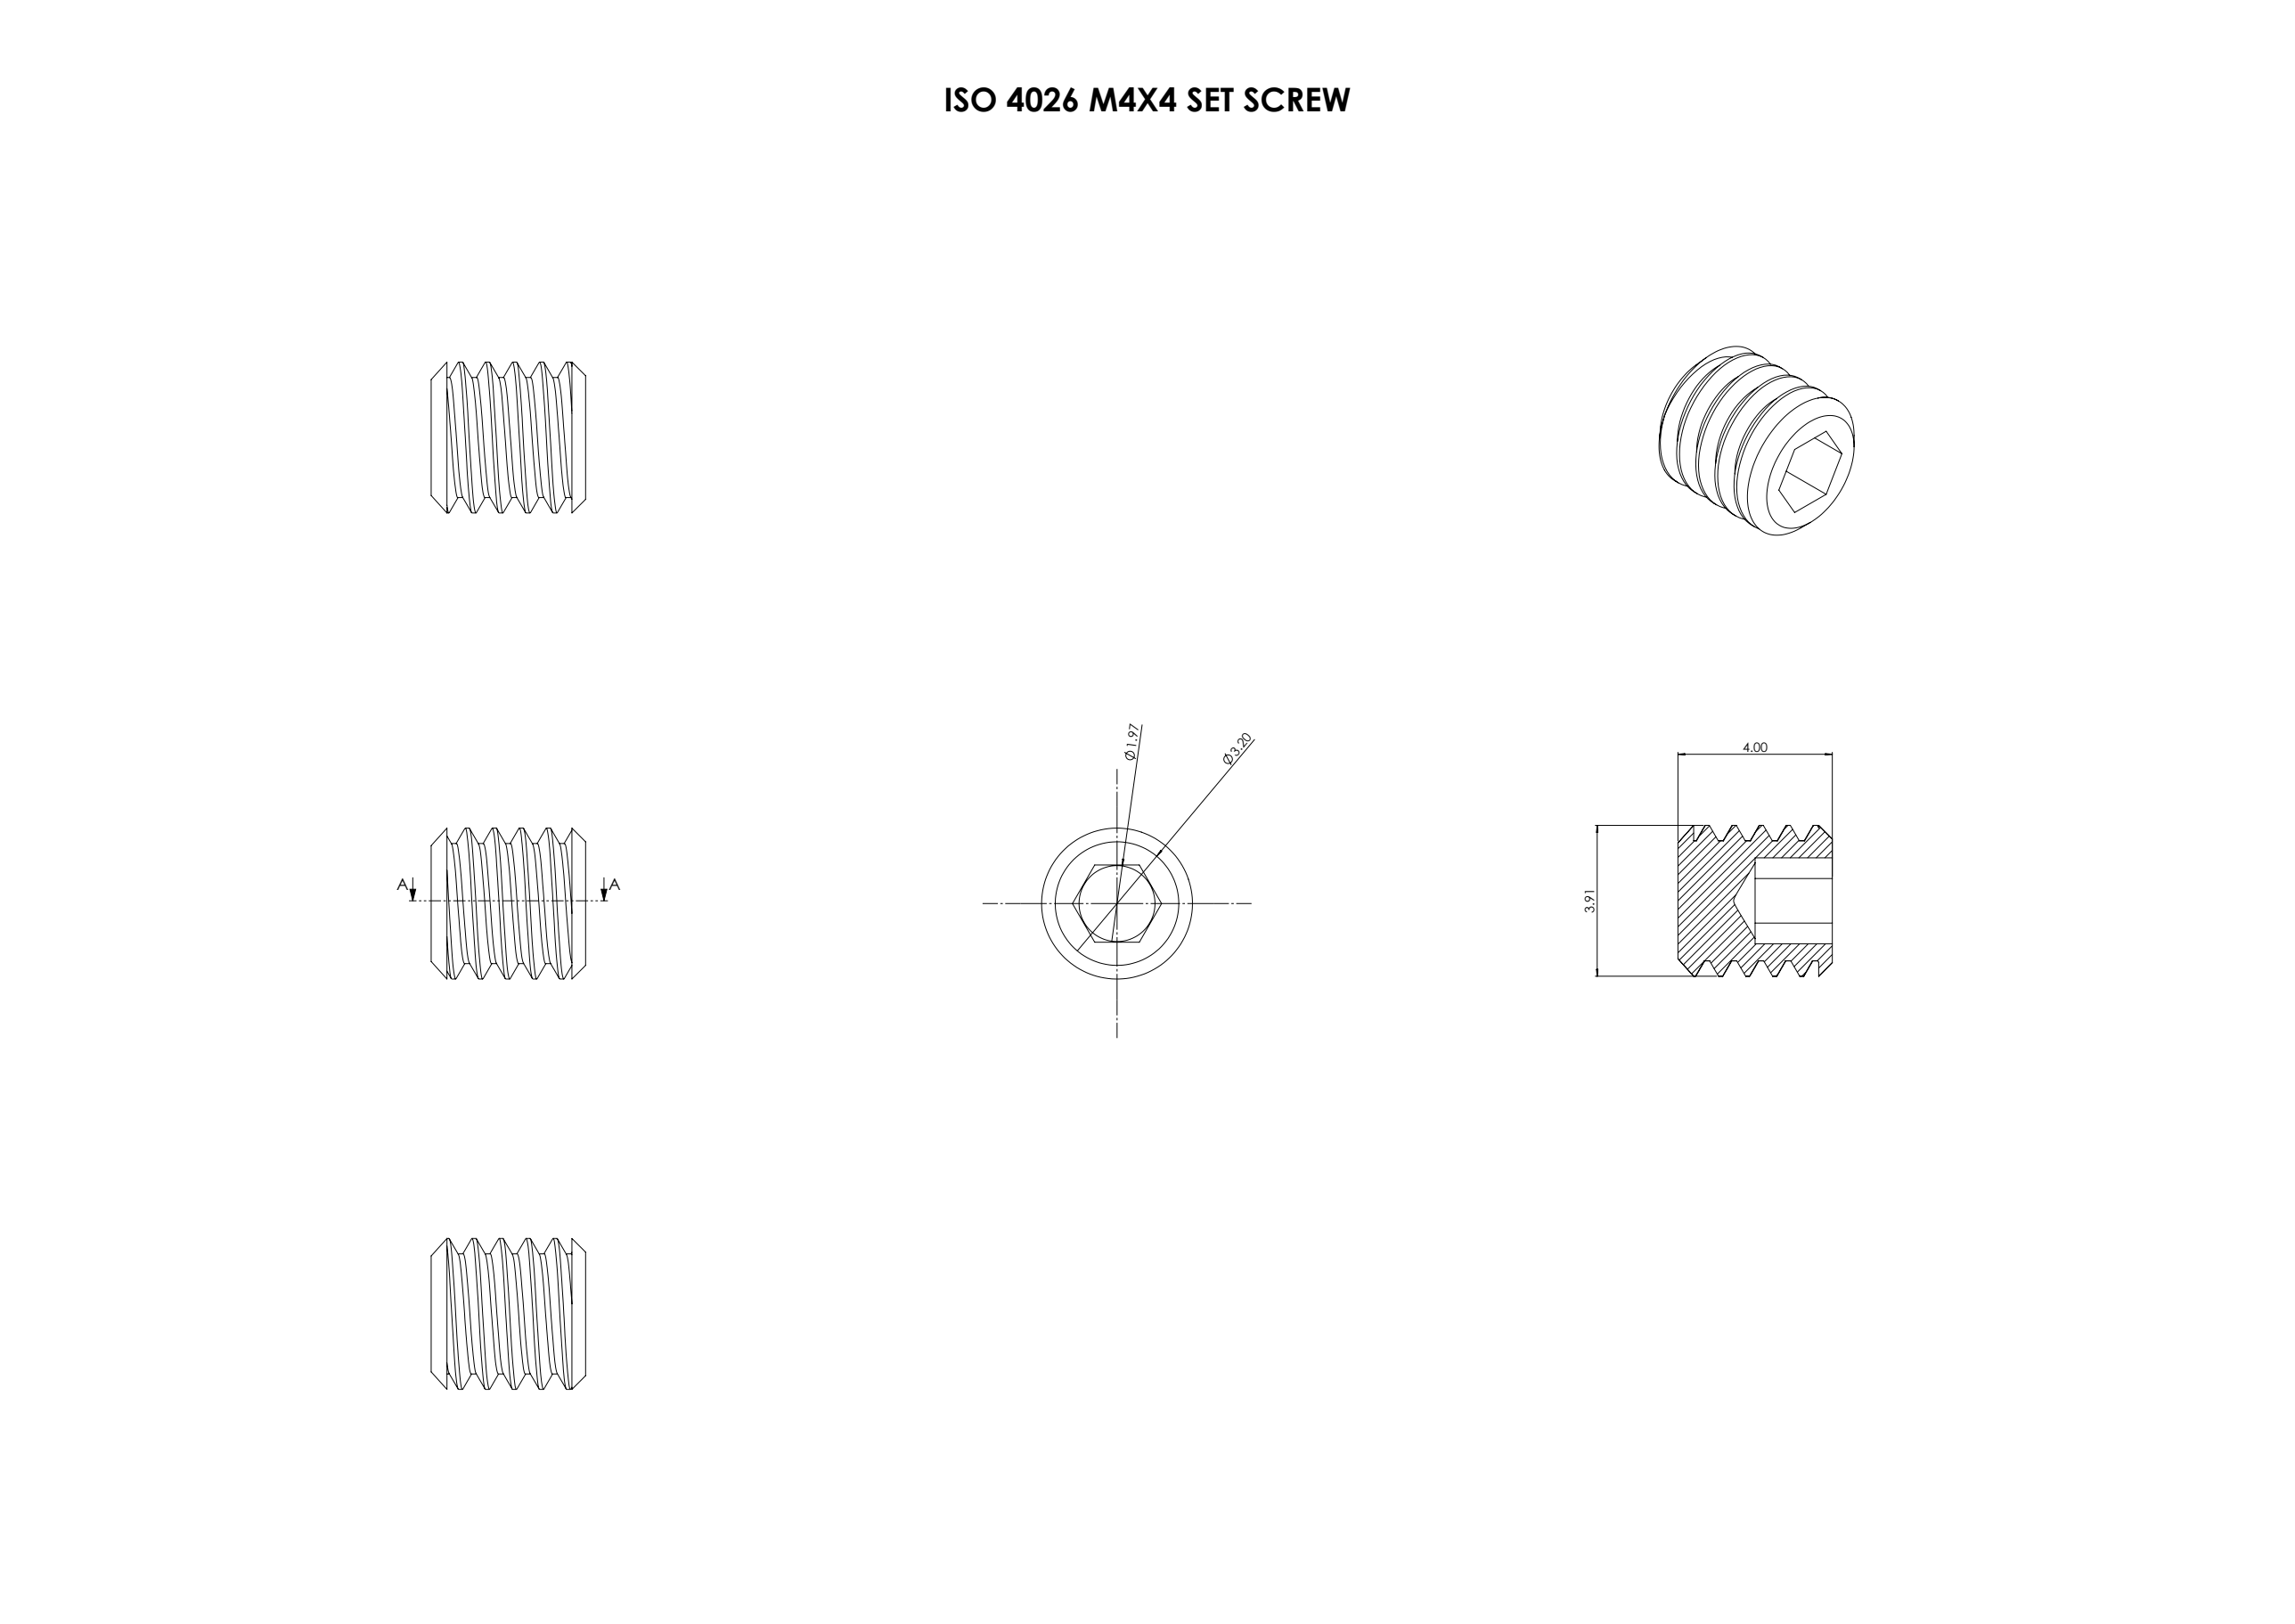
ISO-10303-21;
HEADER;
/* Generated by software containing ST-Developer
 * from STEP Tools, Inc. (www.steptools.com) 
 */

FILE_DESCRIPTION(
/* description */ (''),
/* implementation_level */ '2;1');

FILE_NAME(
/* name */ '09_ISO_4026_M4x4_Set_Screw.step',
/* time_stamp */ '2026-10-11T09:12:28-07:00',
/* author */ (''),
/* organization */ (''),
/* preprocessor_version */ 'ST-DEVELOPER v20.2',
/* originating_system */ 'Autodesk Translation Framework v15.15.0.0',
/* authorisation */ '');

FILE_SCHEMA (('AUTOMOTIVE_DESIGN { 1 0 10303 214 3 1 1 }'));
ENDSEC;

DATA;
#10=MECHANICAL_DESIGN_GEOMETRIC_PRESENTATION_REPRESENTATION('',(#655),#23254);
#173=B_SPLINE_SURFACE_WITH_KNOTS('',3,3,((#22595,#22596,#22597,#22598,#22599,
#22600,#22601,#22602,#22603,#22604,#22605,#22606,#22607,#22608,#22609,#22610,
#22611,#22612,#22613,#22614,#22615,#22616,#22617,#22618,#22619,#22620,#22621,
#22622,#22623,#22624,#22625,#22626,#22627,#22628,#22629),(#22630,#22631,
#22632,#22633,#22634,#22635,#22636,#22637,#22638,#22639,#22640,#22641,#22642,
#22643,#22644,#22645,#22646,#22647,#22648,#22649,#22650,#22651,#22652,#22653,
#22654,#22655,#22656,#22657,#22658,#22659,#22660,#22661,#22662,#22663,#22664),
(#22665,#22666,#22667,#22668,#22669,#22670,#22671,#22672,#22673,#22674,
#22675,#22676,#22677,#22678,#22679,#22680,#22681,#22682,#22683,#22684,#22685,
#22686,#22687,#22688,#22689,#22690,#22691,#22692,#22693,#22694,#22695,#22696,
#22697,#22698,#22699),(#22700,#22701,#22702,#22703,#22704,#22705,#22706,
#22707,#22708,#22709,#22710,#22711,#22712,#22713,#22714,#22715,#22716,#22717,
#22718,#22719,#22720,#22721,#22722,#22723,#22724,#22725,#22726,#22727,#22728,
#22729,#22730,#22731,#22732,#22733,#22734)),.UNSPECIFIED.,.F.,.F.,.F.,(4,
4),(4,1,1,1,1,1,1,1,1,1,1,1,1,1,1,1,1,1,1,1,1,1,1,1,1,1,1,1,1,1,1,1,4),
(0.,0.0460148164544132),(8.31058692273979,9.28321112839862,10.2558353340575,
11.2284595397163,12.2010837453751,13.173707951034,14.1463321566928,15.1189563623516,
16.0915805680104,17.0642047736693,18.0368289793281,19.0094531849869,19.9820773906458,
20.9547015963046,21.9273258019634,22.8999500076223,23.8725742132811,24.8451984189399,
25.8178226245988,26.7904468302576,27.7630710359164,28.7356952415753,29.7083194472341,
30.6809436528929,31.6535678585518,32.6261920642106,33.5988162698694,34.5714404755283,
35.5440646811871,36.5166888868459,37.4893130925048,38.4619372981636,39.4345615038224),
 .UNSPECIFIED.);
#174=B_SPLINE_SURFACE_WITH_KNOTS('',3,3,((#22949,#22950,#22951,#22952,#22953,
#22954,#22955,#22956,#22957,#22958,#22959,#22960,#22961,#22962,#22963,#22964,
#22965,#22966,#22967,#22968,#22969,#22970,#22971,#22972,#22973,#22974,#22975,
#22976,#22977,#22978,#22979,#22980,#22981,#22982,#22983),(#22984,#22985,
#22986,#22987,#22988,#22989,#22990,#22991,#22992,#22993,#22994,#22995,#22996,
#22997,#22998,#22999,#23000,#23001,#23002,#23003,#23004,#23005,#23006,#23007,
#23008,#23009,#23010,#23011,#23012,#23013,#23014,#23015,#23016,#23017,#23018),
(#23019,#23020,#23021,#23022,#23023,#23024,#23025,#23026,#23027,#23028,
#23029,#23030,#23031,#23032,#23033,#23034,#23035,#23036,#23037,#23038,#23039,
#23040,#23041,#23042,#23043,#23044,#23045,#23046,#23047,#23048,#23049,#23050,
#23051,#23052,#23053),(#23054,#23055,#23056,#23057,#23058,#23059,#23060,
#23061,#23062,#23063,#23064,#23065,#23066,#23067,#23068,#23069,#23070,#23071,
#23072,#23073,#23074,#23075,#23076,#23077,#23078,#23079,#23080,#23081,#23082,
#23083,#23084,#23085,#23086,#23087,#23088)),.UNSPECIFIED.,.F.,.F.,.F.,(4,
4),(4,1,1,1,1,1,1,1,1,1,1,1,1,1,1,1,1,1,1,1,1,1,1,1,1,1,1,1,1,1,1,1,4),
(0.,0.0460148164544132),(11.6154215191107,12.5880457247695,13.5606699304283,
14.5332941360872,15.505918341746,16.4785425474048,17.4511667530637,18.4237909587225,
19.3964151643813,20.3690393700402,21.341663575699,22.3142877813578,23.2869119870167,
24.2595361926755,25.2321603983343,26.2047846039932,27.177408809652,28.1500330153108,
29.1226572209696,30.0952814266285,31.0679056322873,32.0405298379462,33.013154043605,
33.9857782492638,34.9584024549226,35.9310266605815,36.9036508662403,37.8762750718991,
38.848899277558,39.8215234832168,40.7941476888756,41.7667718945345,42.7393961001933),
 .UNSPECIFIED.);
#601=B_SPLINE_CURVE_WITH_KNOTS('',3,(#22093,#22094,#22095,#22096,#22097,
#22098,#22099,#22100,#22101,#22102),.UNSPECIFIED.,.F.,.F.,(4,3,3,4),(-4.0925417488383,
-3.89049682263533,-2.9178726169765,-2.0651401332781),.UNSPECIFIED.);
#602=B_SPLINE_CURVE_WITH_KNOTS('',3,(#22105,#22106,#22107,#22108,#22109,
#22110,#22111),.UNSPECIFIED.,.F.,.F.,(4,3,4),(0.,0.972624205658834,1.11419103802959),
 .UNSPECIFIED.);
#603=B_SPLINE_CURVE_WITH_KNOTS('',3,(#22116,#22117,#22118,#22119,#22120,
#22121,#22122,#22123,#22124,#22125,#22126,#22127,#22128,#22129,#22130,#22131,
#22132,#22133,#22134,#22135,#22136,#22137),.UNSPECIFIED.,.F.,.F.,(4,3,3,
3,3,3,3,4),(-10.3757270560179,-9.72624205658833,-8.7536178509295,-7.78099364527067,
-6.80836943961183,-5.835745233953,-4.86312102829416,-4.0925417488383),
 .UNSPECIFIED.);
#604=B_SPLINE_CURVE_WITH_KNOTS('',3,(#22138,#22139,#22140,#22141,#22142,
#22143,#22144,#22145,#22146,#22147,#22148,#22149,#22150,#22151,#22152,#22153,
#22154,#22155,#22156,#22157,#22158,#22159),.UNSPECIFIED.,.F.,.F.,(4,3,3,
3,3,3,3,4),(1.11419103802959,1.94524841131767,2.9178726169765,3.89049682263533,
4.86312102829416,5.835745233953,6.80836943961183,7.39737634520917),
 .UNSPECIFIED.);
#605=B_SPLINE_CURVE_WITH_KNOTS('',3,(#22164,#22165,#22166,#22167,#22168,
#22169,#22170,#22171,#22172,#22173,#22174,#22175,#22176,#22177,#22178,#22179,
#22180,#22181,#22182,#22183,#22184,#22185,#22186,#22187,#22188),
 .UNSPECIFIED.,.F.,.F.,(4,3,3,3,3,3,3,3,4),(-16.6589123631975,-16.5346114962002,
-15.5619872905413,-14.5893630848825,-13.6167388792237,-12.6441146735648,
-11.671490467906,-10.6988662622472,-10.3757270560179),.UNSPECIFIED.);
#606=B_SPLINE_CURVE_WITH_KNOTS('',3,(#22189,#22190,#22191,#22192,#22193,
#22194,#22195,#22196,#22197,#22198,#22199,#22200,#22201,#22202,#22203,#22204,
#22205,#22206,#22207,#22208,#22209,#22210,#22211,#22212,#22213),
 .UNSPECIFIED.,.F.,.F.,(4,3,3,3,3,3,3,3,4),(7.39737634520917,7.78099364527067,
8.7536178509295,9.72624205658833,10.6988662622472,11.671490467906,12.6441146735648,
13.6167388792237,13.6805616523888),.UNSPECIFIED.);
#607=B_SPLINE_CURVE_WITH_KNOTS('',3,(#22218,#22219,#22220,#22221,#22222,
#22223,#22224,#22225,#22226,#22227,#22228,#22229,#22230,#22231,#22232,#22233,
#22234,#22235,#22236,#22237,#22238,#22239),.UNSPECIFIED.,.F.,.F.,(4,3,3,
3,3,3,3,4),(-22.9420976703771,-22.3703567301532,-21.3977325244943,-20.4251083188355,
-19.4524841131767,-18.4798599075178,-17.507235701859,-16.6589123631975),
 .UNSPECIFIED.);
#608=B_SPLINE_CURVE_WITH_KNOTS('',3,(#22240,#22241,#22242,#22243,#22244,
#22245,#22246,#22247,#22248,#22249,#22250,#22251,#22252,#22253,#22254,#22255,
#22256,#22257,#22258,#22259,#22260,#22261),.UNSPECIFIED.,.F.,.F.,(4,3,3,
3,3,3,3,4),(13.6805616523888,14.5893630848825,15.5619872905413,16.5346114962002,
17.507235701859,18.4798599075178,19.4524841131767,19.9637469595683),
 .UNSPECIFIED.);
#609=B_SPLINE_CURVE_WITH_KNOTS('',3,(#22266,#22267,#22268,#22269,#22270,
#22271,#22272,#22273,#22274,#22275,#22276,#22277,#22278,#22279,#22280,#22281,
#22282,#22283,#22284,#22285,#22286,#22287,#22288,#22289,#22290),
 .UNSPECIFIED.,.F.,.F.,(4,3,3,3,3,3,3,3,4),(-29.2252829775566,-29.178726169765,
-28.2061019641061,-27.2334777584473,-26.2608535527885,-25.2882293471297,
-24.3156051414708,-23.342980935812,-22.9420976703771),.UNSPECIFIED.);
#610=B_SPLINE_CURVE_WITH_KNOTS('',3,(#22291,#22292,#22293,#22294,#22295,
#22296,#22297,#22298,#22299,#22300,#22301,#22302,#22303,#22304,#22305,#22306,
#22307,#22308,#22309,#22310,#22311,#22312),.UNSPECIFIED.,.F.,.F.,(4,3,3,
3,3,3,3,4),(19.9637469595683,20.4251083188355,21.3977325244943,22.3703567301532,
23.342980935812,24.3156051414708,25.2882293471297,26.2469322667479),
 .UNSPECIFIED.);
#611=B_SPLINE_CURVE_WITH_KNOTS('',3,(#22318,#22319,#22320,#22321,#22322,
#22323,#22324,#22325,#22326,#22327),.UNSPECIFIED.,.F.,.F.,(4,1,1,1,1,1,
1,4),(34.5575191894877,34.9584024549226,35.9310266605815,36.9036508662403,
37.8762750718991,38.848899277558,39.8215234832168,40.6742559669152),
 .UNSPECIFIED.);
#612=B_SPLINE_CURVE_WITH_KNOTS('',3,(#22330,#22331,#22332,#22333,#22334,
#22335,#22336,#22337,#22338),.UNSPECIFIED.,.F.,.F.,(4,1,1,1,1,1,4),(34.5575191894877,
34.5714404755283,35.5440646811871,36.5166888868459,37.4893130925048,38.4619372981636,
39.4345615038224),.UNSPECIFIED.);
#613=B_SPLINE_CURVE_WITH_KNOTS('',3,(#22343,#22344,#22345,#22346,#22347,
#22348,#22349,#22350,#22351,#22352),.UNSPECIFIED.,.F.,.F.,(4,1,1,1,1,1,
1,4),(28.2743338823081,29.1226572209696,30.0952814266285,31.0679056322873,
32.0405298379462,33.013154043605,33.9857782492638,34.5575191894877),
 .UNSPECIFIED.);
#614=B_SPLINE_CURVE_WITH_KNOTS('',3,(#22353,#22354,#22355,#22356,#22357,
#22358,#22359,#22360,#22361,#22362),.UNSPECIFIED.,.F.,.F.,(4,1,1,1,1,1,
1,4),(28.2743338823081,28.7356952415753,29.7083194472341,30.6809436528929,
31.6535678585518,32.6261920642106,33.5988162698694,34.5575191894877),
 .UNSPECIFIED.);
#615=B_SPLINE_CURVE_WITH_KNOTS('',3,(#22367,#22368,#22369,#22370,#22371,
#22372,#22373,#22374,#22375,#22376,#22377),.UNSPECIFIED.,.F.,.F.,(4,1,1,
1,1,1,1,1,4),(21.9911485751285,22.3142877813578,23.2869119870167,24.2595361926755,
25.2321603983343,26.2047846039932,27.177408809652,28.1500330153108,28.2743338823081),
 .UNSPECIFIED.);
#616=B_SPLINE_CURVE_WITH_KNOTS('',3,(#22378,#22379,#22380,#22381,#22382,
#22383,#22384,#22385,#22386,#22387),.UNSPECIFIED.,.F.,.F.,(4,1,1,1,1,1,
1,4),(21.9911485751285,22.8999500076223,23.8725742132811,24.8451984189399,
25.8178226245988,26.7904468302576,27.7630710359164,28.2743338823081),
 .UNSPECIFIED.);
#617=B_SPLINE_CURVE_WITH_KNOTS('',3,(#22392,#22393,#22394,#22395,#22396,
#22397,#22398,#22399,#22400,#22401),.UNSPECIFIED.,.F.,.F.,(4,1,1,1,1,1,
1,4),(15.707963267949,16.4785425474048,17.4511667530637,18.4237909587225,
19.3964151643813,20.3690393700402,21.341663575699,21.9911485751285),
 .UNSPECIFIED.);
#618=B_SPLINE_CURVE_WITH_KNOTS('',3,(#22402,#22403,#22404,#22405,#22406,
#22407,#22408,#22409,#22410,#22411,#22412),.UNSPECIFIED.,.F.,.F.,(4,1,1,
1,1,1,1,1,4),(15.707963267949,16.0915805680104,17.0642047736693,18.0368289793281,
19.0094531849869,19.9820773906458,20.9547015963046,21.9273258019634,21.9911485751285),
 .UNSPECIFIED.);
#619=B_SPLINE_CURVE_WITH_KNOTS('',3,(#22415,#22416,#22417,#22418,#22419,
#22420,#22421,#22422,#22423,#22424,#22425,#22426,#22427,#22428,#22429,#22430,
#22431,#22432,#22433,#22434,#22435,#22436,#22437,#22438,#22439,#22440,#22441,
#22442,#22443,#22444,#22445,#22446,#22447,#22448,#22449,#22450,#22451,#22452,
#22453,#22454,#22455,#22456,#22457,#22458,#22459,#22460,#22461,#22462,#22463,
#22464,#22465,#22466,#22467,#22468,#22469,#22470,#22471,#22472,#22473,#22474,
#22475,#22476,#22477,#22478,#22479,#22480,#22481,#22482,#22483,#22484,#22485,
#22486,#22487,#22488,#22489,#22490,#22491,#22492,#22493,#22494,#22495,#22496,
#22497,#22498,#22499),.UNSPECIFIED.,.F.,.F.,(4,3,3,3,3,3,3,3,3,3,3,3,3,
3,3,3,3,3,3,3,3,3,3,3,3,3,3,3,4),(-0.366397579005846,-0.347363257188953,
-0.329218211863887,-0.325009393505273,-0.321082490381395,-0.302311388689811,
-0.287356752685602,-0.281279336571668,-0.277587132863102,-0.258196137226557,
-0.238390630512147,-0.224461548048146,-0.216308813318665,-0.212872877173384,
-0.192447164346281,-0.182674300656141,-0.162884351200081,-0.152704079250076,
-0.147209531443036,-0.143832357812886,-0.123380863328339,-0.102495295978267,
-0.0814402231007135,-0.0761230417310904,-0.0722380214272327,-0.0506145254855477,
-0.0289263363699853,-0.00767917833856411,0.),.UNSPECIFIED.);
#620=B_SPLINE_CURVE_WITH_KNOTS('',3,(#22504,#22505,#22506,#22507,#22508,
#22509,#22510,#22511,#22512,#22513,#22514,#22515,#22516,#22517,#22518,#22519,
#22520,#22521,#22522,#22523,#22524,#22525,#22526,#22527,#22528,#22529,#22530,
#22531,#22532,#22533,#22534,#22535,#22536,#22537,#22538,#22539,#22540,#22541,
#22542,#22543,#22544,#22545,#22546,#22547,#22548,#22549,#22550,#22551,#22552,
#22553,#22554,#22555,#22556,#22557,#22558,#22559,#22560,#22561,#22562,#22563,
#22564,#22565,#22566,#22567,#22568,#22569,#22570,#22571,#22572,#22573,#22574,
#22575,#22576,#22577,#22578,#22579,#22580,#22581,#22582,#22583,#22584,#22585,
#22586,#22587,#22588,#22589,#22590,#22591,#22592,#22593,#22594),
 .UNSPECIFIED.,.F.,.F.,(4,3,3,3,3,3,3,3,3,3,3,3,3,3,3,3,3,3,3,3,3,3,3,3,
3,3,3,3,3,3,4),(-0.364629307890671,-0.343563547016126,-0.341292769248738,
-0.318859176467321,-0.313664077314457,-0.309555023850011,-0.288248705342857,
-0.272445620549675,-0.266267591248655,-0.261338548959422,-0.240605115981447,
-0.220331301052625,-0.205704482538819,-0.198406645939577,-0.194091633009513,
-0.190312834535266,-0.170732684798973,-0.161824026997401,-0.141596023622726,
-0.132746272146305,-0.127543418016785,-0.12405868853927,-0.104626158396666,
-0.0852389483794393,-0.0662274169672081,-0.0621520251604476,-0.0589039687159043,
-0.0403067180000117,-0.0220368370756797,-0.00434640786838026,0.),
 .UNSPECIFIED.);
#621=B_SPLINE_CURVE_WITH_KNOTS('',3,(#22735,#22736,#22737,#22738,#22739,
#22740,#22741,#22742,#22743,#22744,#22745,#22746,#22747),.UNSPECIFIED.,
 .F.,.F.,(4,3,3,3,4),(26.2469322667479,26.2608535527885,27.2334777584473,
28.2061019641061,29.0588344478045),.UNSPECIFIED.);
#622=B_SPLINE_CURVE_WITH_KNOTS('',3,(#22749,#22750,#22751,#22752,#22753,
#22754,#22755,#22756,#22757,#22758,#22759,#22760,#22761,#22762,#22763,#22764,
#22765,#22766,#22767,#22768,#22769,#22770,#22771,#22772,#22773,#22774,#22775,
#22776,#22777,#22778,#22779,#22780,#22781,#22782,#22783,#22784,#22785,#22786,
#22787,#22788,#22789,#22790,#22791,#22792,#22793,#22794,#22795,#22796,#22797,
#22798,#22799,#22800,#22801,#22802,#22803,#22804,#22805,#22806,#22807,#22808,
#22809,#22810,#22811,#22812,#22813,#22814,#22815,#22816,#22817,#22818,#22819,
#22820,#22821,#22822,#22823,#22824,#22825,#22826,#22827,#22828,#22829,#22830,
#22831,#22832,#22833),.UNSPECIFIED.,.F.,.F.,(4,3,3,3,3,3,3,3,3,3,3,3,3,
3,3,3,3,3,3,3,3,3,3,3,3,3,3,3,4),(-0.36639757900584,-0.347363257188946,
-0.329218191413008,-0.32500933180285,-0.321082398968414,-0.302311278590842,
-0.287356656349004,-0.281279841150401,-0.277587229488243,-0.258196223178148,
-0.23839071719213,-0.224461613058133,-0.21630881282252,-0.212872875022835,
-0.192447163028057,-0.18267430065614,-0.162884341523524,-0.152704070178304,
-0.147209519148588,-0.143832348410372,-0.123380843105627,-0.102495264673586,
-0.0814401902266025,-0.0761229928137137,-0.0722380376448969,-0.0506145340878939,
-0.0289263495480188,-0.00767922076694763,0.),.UNSPECIFIED.);
#623=B_SPLINE_CURVE_WITH_KNOTS('',3,(#22834,#22835,#22836,#22837,#22838,
#22839,#22840,#22841,#22842),.UNSPECIFIED.,.F.,.F.,(4,1,1,1,1,1,4),(10.3757270560179,
11.2284595397163,12.2010837453751,13.173707951034,14.1463321566928,15.1189563623516,
15.707963267949),.UNSPECIFIED.);
#624=B_SPLINE_CURVE_WITH_KNOTS('',3,(#22848,#22849,#22850,#22851,#22852,
#22853,#22854,#22855,#22856,#22857,#22858,#22859,#22860,#22861,#22862,#22863,
#22864,#22865,#22866,#22867,#22868,#22869,#22870,#22871,#22872,#22873,#22874,
#22875,#22876,#22877,#22878,#22879,#22880,#22881,#22882,#22883,#22884,#22885,
#22886,#22887,#22888,#22889,#22890,#22891,#22892,#22893,#22894,#22895,#22896,
#22897,#22898,#22899,#22900,#22901,#22902,#22903,#22904,#22905,#22906,#22907,
#22908,#22909,#22910,#22911,#22912,#22913,#22914,#22915,#22916,#22917,#22918,
#22919,#22920,#22921,#22922,#22923,#22924,#22925,#22926,#22927,#22928,#22929,
#22930,#22931,#22932,#22933,#22934,#22935,#22936,#22937,#22938),
 .UNSPECIFIED.,.F.,.F.,(4,3,3,3,3,3,3,3,3,3,3,3,3,3,3,3,3,3,3,3,3,3,3,3,
3,3,3,3,3,3,4),(-0.364629307890668,-0.343563554406758,-0.341292769248734,
-0.318859176467317,-0.313664088958277,-0.309555028947178,-0.288248710841805,
-0.272445625361255,-0.266267609571851,-0.26133855187035,-0.240605120999503,
-0.220331326646483,-0.205704501734212,-0.198406690155409,-0.194092634197369,
-0.190313011659516,-0.170732881684786,-0.161824026997401,-0.141596023622726,
-0.132746272146305,-0.127543414865392,-0.124058687169216,-0.104626163550009,
-0.0852389404586007,-0.0662273798318025,-0.06215172276271,-0.0589034837300999,
-0.0403062183939592,-0.0220363157458943,-0.00434585567455788,0.),
 .UNSPECIFIED.);
#625=B_SPLINE_CURVE_WITH_KNOTS('',3,(#22941,#22942,#22943,#22944,#22945,
#22946,#22947,#22948),.UNSPECIFIED.,.F.,.F.,(4,1,1,1,1,4),(11.6154215191107,
12.5880457247695,13.5606699304283,14.5332941360872,15.505918341746,15.707963267949),
 .UNSPECIFIED.);
#626=B_SPLINE_CURVE_WITH_KNOTS('',3,(#23089,#23090,#23091,#23092,#23093,
#23094,#23095),.UNSPECIFIED.,.F.,.F.,(4,3,4),(-31.1239745810827,-30.1513503754238,
-29.2252829775566),.UNSPECIFIED.);
#635=SHAPE_REPRESENTATION_RELATIONSHIP('SRR','None',#23308,#645);
#645=ADVANCED_BREP_SHAPE_REPRESENTATION('',(#665),#23252);
#655=STYLED_ITEM('',(#23469),#665);
#665=MANIFOLD_SOLID_BREP('Body1',#7033);
#756=CONICAL_SURFACE('',#7775,0.5,1.02305631307899);
#757=CONICAL_SURFACE('',#7786,1.75,0.83798122500839);
#758=CONICAL_SURFACE('',#7789,1.8,0.785398163397448);
#846=FACE_BOUND('',#1818,.T.);
#847=FACE_BOUND('',#1824,.T.);
#960=PLANE('',#7767);
#961=PLANE('',#7770);
#962=PLANE('',#7777);
#963=PLANE('',#7778);
#964=PLANE('',#7779);
#965=PLANE('',#7780);
#966=PLANE('',#7781);
#967=PLANE('',#7782);
#968=PLANE('',#7783);
#969=PLANE('',#7784);
#970=PLANE('',#7791);
#1335=FACE_OUTER_BOUND('',#1796,.T.);
#1336=FACE_OUTER_BOUND('',#1797,.T.);
#1337=FACE_OUTER_BOUND('',#1798,.T.);
#1338=FACE_OUTER_BOUND('',#1799,.T.);
#1339=FACE_OUTER_BOUND('',#1800,.T.);
#1340=FACE_OUTER_BOUND('',#1801,.T.);
#1341=FACE_OUTER_BOUND('',#1802,.T.);
#1342=FACE_OUTER_BOUND('',#1803,.T.);
#1343=FACE_OUTER_BOUND('',#1804,.T.);
#1344=FACE_OUTER_BOUND('',#1805,.T.);
#1345=FACE_OUTER_BOUND('',#1806,.T.);
#1346=FACE_OUTER_BOUND('',#1807,.T.);
#1347=FACE_OUTER_BOUND('',#1808,.T.);
#1348=FACE_OUTER_BOUND('',#1809,.T.);
#1349=FACE_OUTER_BOUND('',#1810,.T.);
#1350=FACE_OUTER_BOUND('',#1811,.T.);
#1351=FACE_OUTER_BOUND('',#1812,.T.);
#1352=FACE_OUTER_BOUND('',#1813,.T.);
#1353=FACE_OUTER_BOUND('',#1814,.T.);
#1354=FACE_OUTER_BOUND('',#1815,.T.);
#1355=FACE_OUTER_BOUND('',#1816,.T.);
#1356=FACE_OUTER_BOUND('',#1817,.T.);
#1357=FACE_OUTER_BOUND('',#1819,.T.);
#1358=FACE_OUTER_BOUND('',#1820,.T.);
#1359=FACE_OUTER_BOUND('',#1821,.T.);
#1360=FACE_OUTER_BOUND('',#1822,.T.);
#1361=FACE_OUTER_BOUND('',#1823,.T.);
#1796=EDGE_LOOP('',(#6373,#6374,#6375,#6376));
#1797=EDGE_LOOP('',(#6377,#6378,#6379,#6380));
#1798=EDGE_LOOP('',(#6381,#6382,#6383,#6384));
#1799=EDGE_LOOP('',(#6385,#6386,#6387,#6388));
#1800=EDGE_LOOP('',(#6389,#6390,#6391,#6392));
#1801=EDGE_LOOP('',(#6393,#6394,#6395,#6396));
#1802=EDGE_LOOP('',(#6397,#6398,#6399,#6400));
#1803=EDGE_LOOP('',(#6401,#6402,#6403,#6404));
#1804=EDGE_LOOP('',(#6405,#6406,#6407,#6408));
#1805=EDGE_LOOP('',(#6409,#6410,#6411,#6412,#6413));
#1806=EDGE_LOOP('',(#6414,#6415,#6416,#6417,#6418,#6419,#6420,#6421,#6422,
#6423,#6424,#6425,#6426));
#1807=EDGE_LOOP('',(#6427,#6428,#6429,#6430,#6431));
#1808=EDGE_LOOP('',(#6432,#6433,#6434,#6435));
#1809=EDGE_LOOP('',(#6436,#6437,#6438,#6439,#6440,#6441,#6442,#6443,#6444,
#6445,#6446,#6447,#6448));
#1810=EDGE_LOOP('',(#6449,#6450,#6451));
#1811=EDGE_LOOP('',(#6452,#6453,#6454,#6455));
#1812=EDGE_LOOP('',(#6456,#6457,#6458,#6459));
#1813=EDGE_LOOP('',(#6460,#6461,#6462,#6463));
#1814=EDGE_LOOP('',(#6464,#6465,#6466,#6467));
#1815=EDGE_LOOP('',(#6468,#6469,#6470,#6471));
#1816=EDGE_LOOP('',(#6472,#6473,#6474,#6475));
#1817=EDGE_LOOP('',(#6476,#6477,#6478,#6479,#6480,#6481));
#1818=EDGE_LOOP('',(#6482));
#1819=EDGE_LOOP('',(#6483));
#1820=EDGE_LOOP('',(#6484,#6485,#6486,#6487,#6488,#6489));
#1821=EDGE_LOOP('',(#6490,#6491,#6492,#6493));
#1822=EDGE_LOOP('',(#6494,#6495,#6496,#6497,#6498,#6499));
#1823=EDGE_LOOP('',(#6500));
#1824=EDGE_LOOP('',(#6501,#6502,#6503,#6504,#6505,#6506));
#2048=LINE('',#22091,#2307);
#2049=LINE('',#22115,#2308);
#2050=LINE('',#22163,#2309);
#2051=LINE('',#22217,#2310);
#2052=LINE('',#22265,#2311);
#2053=LINE('',#22316,#2312);
#2054=LINE('',#22342,#2313);
#2055=LINE('',#22366,#2314);
#2056=LINE('',#22391,#2315);
#2057=LINE('',#23099,#2316);
#2058=LINE('',#23104,#2317);
#2059=LINE('',#23106,#2318);
#2060=LINE('',#23108,#2319);
#2061=LINE('',#23109,#2320);
#2062=LINE('',#23112,#2321);
#2063=LINE('',#23114,#2322);
#2064=LINE('',#23115,#2323);
#2065=LINE('',#23118,#2324);
#2066=LINE('',#23120,#2325);
#2067=LINE('',#23121,#2326);
#2068=LINE('',#23124,#2327);
#2069=LINE('',#23126,#2328);
#2070=LINE('',#23127,#2329);
#2071=LINE('',#23130,#2330);
#2072=LINE('',#23132,#2331);
#2073=LINE('',#23133,#2332);
#2074=LINE('',#23135,#2333);
#2075=LINE('',#23136,#2334);
#2076=LINE('',#23142,#2335);
#2077=LINE('',#23148,#2336);
#2307=VECTOR('',#9260,2.);
#2308=VECTOR('',#9265,2.);
#2309=VECTOR('',#9268,2.);
#2310=VECTOR('',#9271,2.);
#2311=VECTOR('',#9274,2.);
#2312=VECTOR('',#9277,1.5555);
#2313=VECTOR('',#9282,1.5555);
#2314=VECTOR('',#9285,1.5555);
#2315=VECTOR('',#9288,1.5555);
#2316=VECTOR('',#9307,0.5);
#2317=VECTOR('',#9312,10.);
#2318=VECTOR('',#9313,10.);
#2319=VECTOR('',#9314,10.);
#2320=VECTOR('',#9315,10.);
#2321=VECTOR('',#9318,10.);
#2322=VECTOR('',#9319,10.);
#2323=VECTOR('',#9320,10.);
#2324=VECTOR('',#9323,10.);
#2325=VECTOR('',#9324,10.);
#2326=VECTOR('',#9325,10.);
#2327=VECTOR('',#9328,10.);
#2328=VECTOR('',#9329,10.);
#2329=VECTOR('',#9330,10.);
#2330=VECTOR('',#9333,10.);
#2331=VECTOR('',#9334,10.);
#2332=VECTOR('',#9335,10.);
#2333=VECTOR('',#9338,10.);
#2334=VECTOR('',#9339,10.);
#2335=VECTOR('',#9348,1.75);
#2336=VECTOR('',#9357,1.8);
#2683=CIRCLE('',#7757,1.954);
#2684=CIRCLE('',#7763,1.5555);
#2685=CIRCLE('',#7768,1.954);
#2686=CIRCLE('',#7769,1.954);
#2687=CIRCLE('',#7771,1.954);
#2688=CIRCLE('',#7772,1.954);
#2689=CIRCLE('',#7773,1.5555);
#2690=CIRCLE('',#7776,0.98360655737705);
#2691=CIRCLE('',#7785,1.5);
#2692=CIRCLE('',#7788,1.954);
#2693=CIRCLE('',#7790,1.6);
#3341=VERTEX_POINT('',#22089);
#3342=VERTEX_POINT('',#22090);
#3343=VERTEX_POINT('',#22092);
#3344=VERTEX_POINT('',#22103);
#3345=VERTEX_POINT('',#22113);
#3346=VERTEX_POINT('',#22114);
#3347=VERTEX_POINT('',#22161);
#3348=VERTEX_POINT('',#22162);
#3349=VERTEX_POINT('',#22215);
#3350=VERTEX_POINT('',#22216);
#3351=VERTEX_POINT('',#22263);
#3352=VERTEX_POINT('',#22264);
#3353=VERTEX_POINT('',#22314);
#3354=VERTEX_POINT('',#22315);
#3355=VERTEX_POINT('',#22317);
#3356=VERTEX_POINT('',#22328);
#3357=VERTEX_POINT('',#22340);
#3358=VERTEX_POINT('',#22341);
#3359=VERTEX_POINT('',#22364);
#3360=VERTEX_POINT('',#22365);
#3361=VERTEX_POINT('',#22389);
#3362=VERTEX_POINT('',#22390);
#3363=VERTEX_POINT('',#22414);
#3364=VERTEX_POINT('',#22500);
#3365=VERTEX_POINT('',#22502);
#3366=VERTEX_POINT('',#22748);
#3367=VERTEX_POINT('',#22844);
#3368=VERTEX_POINT('',#22847);
#3369=VERTEX_POINT('',#23097);
#3370=VERTEX_POINT('',#23098);
#3371=VERTEX_POINT('',#23102);
#3372=VERTEX_POINT('',#23103);
#3373=VERTEX_POINT('',#23105);
#3374=VERTEX_POINT('',#23107);
#3375=VERTEX_POINT('',#23111);
#3376=VERTEX_POINT('',#23113);
#3377=VERTEX_POINT('',#23117);
#3378=VERTEX_POINT('',#23119);
#3379=VERTEX_POINT('',#23123);
#3380=VERTEX_POINT('',#23125);
#3381=VERTEX_POINT('',#23129);
#3382=VERTEX_POINT('',#23131);
#3383=VERTEX_POINT('',#23139);
#3384=VERTEX_POINT('',#23146);
#4362=EDGE_CURVE('',#3341,#3342,#2048,.T.);
#4363=EDGE_CURVE('',#3341,#3343,#601,.T.);
#4364=EDGE_CURVE('',#3343,#3344,#2683,.T.);
#4365=EDGE_CURVE('',#3344,#3342,#602,.T.);
#4366=EDGE_CURVE('',#3345,#3346,#2049,.T.);
#4367=EDGE_CURVE('',#3345,#3341,#603,.T.);
#4368=EDGE_CURVE('',#3342,#3346,#604,.T.);
#4369=EDGE_CURVE('',#3347,#3348,#2050,.T.);
#4370=EDGE_CURVE('',#3347,#3345,#605,.T.);
#4371=EDGE_CURVE('',#3346,#3348,#606,.T.);
#4372=EDGE_CURVE('',#3349,#3350,#2051,.T.);
#4373=EDGE_CURVE('',#3349,#3347,#607,.T.);
#4374=EDGE_CURVE('',#3348,#3350,#608,.T.);
#4375=EDGE_CURVE('',#3351,#3352,#2052,.T.);
#4376=EDGE_CURVE('',#3351,#3349,#609,.T.);
#4377=EDGE_CURVE('',#3350,#3352,#610,.T.);
#4378=EDGE_CURVE('',#3353,#3354,#2053,.T.);
#4379=EDGE_CURVE('',#3353,#3355,#611,.T.);
#4380=EDGE_CURVE('',#3356,#3355,#2684,.T.);
#4381=EDGE_CURVE('',#3354,#3356,#612,.T.);
#4382=EDGE_CURVE('',#3357,#3358,#2054,.T.);
#4383=EDGE_CURVE('',#3357,#3353,#613,.T.);
#4384=EDGE_CURVE('',#3358,#3354,#614,.T.);
#4385=EDGE_CURVE('',#3359,#3360,#2055,.T.);
#4386=EDGE_CURVE('',#3359,#3357,#615,.T.);
#4387=EDGE_CURVE('',#3360,#3358,#616,.T.);
#4388=EDGE_CURVE('',#3361,#3362,#2056,.T.);
#4389=EDGE_CURVE('',#3361,#3359,#617,.T.);
#4390=EDGE_CURVE('',#3362,#3360,#618,.T.);
#4391=EDGE_CURVE('',#3355,#3363,#619,.T.);
#4392=EDGE_CURVE('',#3364,#3363,#2685,.F.);
#4393=EDGE_CURVE('',#3365,#3364,#2686,.F.);
#4394=EDGE_CURVE('',#3365,#3356,#620,.T.);
#4395=EDGE_CURVE('',#3352,#3365,#621,.T.);
#4396=EDGE_CURVE('',#3366,#3344,#622,.T.);
#4397=EDGE_CURVE('',#3366,#3362,#623,.T.);
#4398=EDGE_CURVE('',#3344,#3367,#2687,.T.);
#4399=EDGE_CURVE('',#3367,#3343,#2688,.T.);
#4400=EDGE_CURVE('',#3343,#3368,#624,.T.);
#4401=EDGE_CURVE('',#3368,#3366,#2689,.T.);
#4402=EDGE_CURVE('',#3368,#3361,#625,.T.);
#4403=EDGE_CURVE('',#3363,#3351,#626,.T.);
#4404=EDGE_CURVE('',#3369,#3370,#2057,.T.);
#4405=EDGE_CURVE('',#3370,#3370,#2690,.T.);
#4406=EDGE_CURVE('',#3371,#3372,#2058,.T.);
#4407=EDGE_CURVE('',#3373,#3371,#2059,.T.);
#4408=EDGE_CURVE('',#3374,#3373,#2060,.T.);
#4409=EDGE_CURVE('',#3374,#3372,#2061,.T.);
#4410=EDGE_CURVE('',#3372,#3375,#2062,.T.);
#4411=EDGE_CURVE('',#3376,#3374,#2063,.T.);
#4412=EDGE_CURVE('',#3376,#3375,#2064,.T.);
#4413=EDGE_CURVE('',#3375,#3377,#2065,.T.);
#4414=EDGE_CURVE('',#3378,#3376,#2066,.T.);
#4415=EDGE_CURVE('',#3378,#3377,#2067,.T.);
#4416=EDGE_CURVE('',#3377,#3379,#2068,.T.);
#4417=EDGE_CURVE('',#3380,#3378,#2069,.T.);
#4418=EDGE_CURVE('',#3380,#3379,#2070,.T.);
#4419=EDGE_CURVE('',#3379,#3381,#2071,.T.);
#4420=EDGE_CURVE('',#3382,#3380,#2072,.T.);
#4421=EDGE_CURVE('',#3382,#3381,#2073,.T.);
#4422=EDGE_CURVE('',#3381,#3371,#2074,.T.);
#4423=EDGE_CURVE('',#3373,#3382,#2075,.T.);
#4424=EDGE_CURVE('',#3383,#3383,#2691,.T.);
#4425=EDGE_CURVE('',#3367,#3383,#2076,.T.);
#4426=EDGE_CURVE('',#3363,#3365,#2692,.F.);
#4427=EDGE_CURVE('',#3384,#3384,#2693,.T.);
#4428=EDGE_CURVE('',#3384,#3364,#2077,.T.);
#6373=ORIENTED_EDGE('',*,*,#4362,.F.);
#6374=ORIENTED_EDGE('',*,*,#4363,.T.);
#6375=ORIENTED_EDGE('',*,*,#4364,.T.);
#6376=ORIENTED_EDGE('',*,*,#4365,.T.);
#6377=ORIENTED_EDGE('',*,*,#4366,.F.);
#6378=ORIENTED_EDGE('',*,*,#4367,.T.);
#6379=ORIENTED_EDGE('',*,*,#4362,.T.);
#6380=ORIENTED_EDGE('',*,*,#4368,.T.);
#6381=ORIENTED_EDGE('',*,*,#4369,.F.);
#6382=ORIENTED_EDGE('',*,*,#4370,.T.);
#6383=ORIENTED_EDGE('',*,*,#4366,.T.);
#6384=ORIENTED_EDGE('',*,*,#4371,.T.);
#6385=ORIENTED_EDGE('',*,*,#4372,.F.);
#6386=ORIENTED_EDGE('',*,*,#4373,.T.);
#6387=ORIENTED_EDGE('',*,*,#4369,.T.);
#6388=ORIENTED_EDGE('',*,*,#4374,.T.);
#6389=ORIENTED_EDGE('',*,*,#4375,.F.);
#6390=ORIENTED_EDGE('',*,*,#4376,.T.);
#6391=ORIENTED_EDGE('',*,*,#4372,.T.);
#6392=ORIENTED_EDGE('',*,*,#4377,.T.);
#6393=ORIENTED_EDGE('',*,*,#4378,.F.);
#6394=ORIENTED_EDGE('',*,*,#4379,.T.);
#6395=ORIENTED_EDGE('',*,*,#4380,.F.);
#6396=ORIENTED_EDGE('',*,*,#4381,.F.);
#6397=ORIENTED_EDGE('',*,*,#4382,.F.);
#6398=ORIENTED_EDGE('',*,*,#4383,.T.);
#6399=ORIENTED_EDGE('',*,*,#4378,.T.);
#6400=ORIENTED_EDGE('',*,*,#4384,.F.);
#6401=ORIENTED_EDGE('',*,*,#4385,.F.);
#6402=ORIENTED_EDGE('',*,*,#4386,.T.);
#6403=ORIENTED_EDGE('',*,*,#4382,.T.);
#6404=ORIENTED_EDGE('',*,*,#4387,.F.);
#6405=ORIENTED_EDGE('',*,*,#4388,.F.);
#6406=ORIENTED_EDGE('',*,*,#4389,.T.);
#6407=ORIENTED_EDGE('',*,*,#4385,.T.);
#6408=ORIENTED_EDGE('',*,*,#4390,.F.);
#6409=ORIENTED_EDGE('',*,*,#4380,.T.);
#6410=ORIENTED_EDGE('',*,*,#4391,.T.);
#6411=ORIENTED_EDGE('',*,*,#4392,.F.);
#6412=ORIENTED_EDGE('',*,*,#4393,.F.);
#6413=ORIENTED_EDGE('',*,*,#4394,.T.);
#6414=ORIENTED_EDGE('',*,*,#4394,.F.);
#6415=ORIENTED_EDGE('',*,*,#4395,.F.);
#6416=ORIENTED_EDGE('',*,*,#4377,.F.);
#6417=ORIENTED_EDGE('',*,*,#4374,.F.);
#6418=ORIENTED_EDGE('',*,*,#4371,.F.);
#6419=ORIENTED_EDGE('',*,*,#4368,.F.);
#6420=ORIENTED_EDGE('',*,*,#4365,.F.);
#6421=ORIENTED_EDGE('',*,*,#4396,.F.);
#6422=ORIENTED_EDGE('',*,*,#4397,.T.);
#6423=ORIENTED_EDGE('',*,*,#4390,.T.);
#6424=ORIENTED_EDGE('',*,*,#4387,.T.);
#6425=ORIENTED_EDGE('',*,*,#4384,.T.);
#6426=ORIENTED_EDGE('',*,*,#4381,.T.);
#6427=ORIENTED_EDGE('',*,*,#4398,.T.);
#6428=ORIENTED_EDGE('',*,*,#4399,.T.);
#6429=ORIENTED_EDGE('',*,*,#4400,.T.);
#6430=ORIENTED_EDGE('',*,*,#4401,.T.);
#6431=ORIENTED_EDGE('',*,*,#4396,.T.);
#6432=ORIENTED_EDGE('',*,*,#4388,.T.);
#6433=ORIENTED_EDGE('',*,*,#4397,.F.);
#6434=ORIENTED_EDGE('',*,*,#4401,.F.);
#6435=ORIENTED_EDGE('',*,*,#4402,.T.);
#6436=ORIENTED_EDGE('',*,*,#4391,.F.);
#6437=ORIENTED_EDGE('',*,*,#4379,.F.);
#6438=ORIENTED_EDGE('',*,*,#4383,.F.);
#6439=ORIENTED_EDGE('',*,*,#4386,.F.);
#6440=ORIENTED_EDGE('',*,*,#4389,.F.);
#6441=ORIENTED_EDGE('',*,*,#4402,.F.);
#6442=ORIENTED_EDGE('',*,*,#4400,.F.);
#6443=ORIENTED_EDGE('',*,*,#4363,.F.);
#6444=ORIENTED_EDGE('',*,*,#4367,.F.);
#6445=ORIENTED_EDGE('',*,*,#4370,.F.);
#6446=ORIENTED_EDGE('',*,*,#4373,.F.);
#6447=ORIENTED_EDGE('',*,*,#4376,.F.);
#6448=ORIENTED_EDGE('',*,*,#4403,.F.);
#6449=ORIENTED_EDGE('',*,*,#4404,.T.);
#6450=ORIENTED_EDGE('',*,*,#4405,.F.);
#6451=ORIENTED_EDGE('',*,*,#4404,.F.);
#6452=ORIENTED_EDGE('',*,*,#4406,.F.);
#6453=ORIENTED_EDGE('',*,*,#4407,.F.);
#6454=ORIENTED_EDGE('',*,*,#4408,.F.);
#6455=ORIENTED_EDGE('',*,*,#4409,.T.);
#6456=ORIENTED_EDGE('',*,*,#4410,.F.);
#6457=ORIENTED_EDGE('',*,*,#4409,.F.);
#6458=ORIENTED_EDGE('',*,*,#4411,.F.);
#6459=ORIENTED_EDGE('',*,*,#4412,.T.);
#6460=ORIENTED_EDGE('',*,*,#4413,.F.);
#6461=ORIENTED_EDGE('',*,*,#4412,.F.);
#6462=ORIENTED_EDGE('',*,*,#4414,.F.);
#6463=ORIENTED_EDGE('',*,*,#4415,.T.);
#6464=ORIENTED_EDGE('',*,*,#4416,.F.);
#6465=ORIENTED_EDGE('',*,*,#4415,.F.);
#6466=ORIENTED_EDGE('',*,*,#4417,.F.);
#6467=ORIENTED_EDGE('',*,*,#4418,.T.);
#6468=ORIENTED_EDGE('',*,*,#4419,.F.);
#6469=ORIENTED_EDGE('',*,*,#4418,.F.);
#6470=ORIENTED_EDGE('',*,*,#4420,.F.);
#6471=ORIENTED_EDGE('',*,*,#4421,.T.);
#6472=ORIENTED_EDGE('',*,*,#4422,.F.);
#6473=ORIENTED_EDGE('',*,*,#4421,.F.);
#6474=ORIENTED_EDGE('',*,*,#4423,.F.);
#6475=ORIENTED_EDGE('',*,*,#4407,.T.);
#6476=ORIENTED_EDGE('',*,*,#4414,.T.);
#6477=ORIENTED_EDGE('',*,*,#4411,.T.);
#6478=ORIENTED_EDGE('',*,*,#4408,.T.);
#6479=ORIENTED_EDGE('',*,*,#4423,.T.);
#6480=ORIENTED_EDGE('',*,*,#4420,.T.);
#6481=ORIENTED_EDGE('',*,*,#4417,.T.);
#6482=ORIENTED_EDGE('',*,*,#4405,.T.);
#6483=ORIENTED_EDGE('',*,*,#4424,.F.);
#6484=ORIENTED_EDGE('',*,*,#4398,.F.);
#6485=ORIENTED_EDGE('',*,*,#4364,.F.);
#6486=ORIENTED_EDGE('',*,*,#4399,.F.);
#6487=ORIENTED_EDGE('',*,*,#4425,.T.);
#6488=ORIENTED_EDGE('',*,*,#4424,.T.);
#6489=ORIENTED_EDGE('',*,*,#4425,.F.);
#6490=ORIENTED_EDGE('',*,*,#4375,.T.);
#6491=ORIENTED_EDGE('',*,*,#4395,.T.);
#6492=ORIENTED_EDGE('',*,*,#4426,.F.);
#6493=ORIENTED_EDGE('',*,*,#4403,.T.);
#6494=ORIENTED_EDGE('',*,*,#4427,.F.);
#6495=ORIENTED_EDGE('',*,*,#4428,.T.);
#6496=ORIENTED_EDGE('',*,*,#4392,.T.);
#6497=ORIENTED_EDGE('',*,*,#4426,.T.);
#6498=ORIENTED_EDGE('',*,*,#4393,.T.);
#6499=ORIENTED_EDGE('',*,*,#4428,.F.);
#6500=ORIENTED_EDGE('',*,*,#4427,.T.);
#6501=ORIENTED_EDGE('',*,*,#4416,.T.);
#6502=ORIENTED_EDGE('',*,*,#4419,.T.);
#6503=ORIENTED_EDGE('',*,*,#4422,.T.);
#6504=ORIENTED_EDGE('',*,*,#4406,.T.);
#6505=ORIENTED_EDGE('',*,*,#4410,.T.);
#6506=ORIENTED_EDGE('',*,*,#4413,.T.);
#6615=CYLINDRICAL_SURFACE('',#7756,1.954);
#6616=CYLINDRICAL_SURFACE('',#7758,1.954);
#6617=CYLINDRICAL_SURFACE('',#7759,1.954);
#6618=CYLINDRICAL_SURFACE('',#7760,1.954);
#6619=CYLINDRICAL_SURFACE('',#7761,1.954);
#6620=CYLINDRICAL_SURFACE('',#7762,1.5555);
#6621=CYLINDRICAL_SURFACE('',#7764,1.5555);
#6622=CYLINDRICAL_SURFACE('',#7765,1.5555);
#6623=CYLINDRICAL_SURFACE('',#7766,1.5555);
#6624=CYLINDRICAL_SURFACE('',#7774,1.5555);
#6625=CYLINDRICAL_SURFACE('',#7787,1.954);
#6986=ADVANCED_FACE('',(#1335),#6615,.T.);
#6987=ADVANCED_FACE('',(#1336),#6616,.T.);
#6988=ADVANCED_FACE('',(#1337),#6617,.T.);
#6989=ADVANCED_FACE('',(#1338),#6618,.T.);
#6990=ADVANCED_FACE('',(#1339),#6619,.T.);
#6991=ADVANCED_FACE('',(#1340),#6620,.T.);
#6992=ADVANCED_FACE('',(#1341),#6621,.T.);
#6993=ADVANCED_FACE('',(#1342),#6622,.T.);
#6994=ADVANCED_FACE('',(#1343),#6623,.T.);
#6995=ADVANCED_FACE('',(#1344),#960,.F.);
#6996=ADVANCED_FACE('',(#1345),#173,.F.);
#6997=ADVANCED_FACE('',(#1346),#961,.T.);
#6998=ADVANCED_FACE('',(#1347),#6624,.T.);
#6999=ADVANCED_FACE('',(#1348),#174,.F.);
#7000=ADVANCED_FACE('',(#1349),#756,.F.);
#7001=ADVANCED_FACE('',(#1350),#962,.F.);
#7002=ADVANCED_FACE('',(#1351),#963,.F.);
#7003=ADVANCED_FACE('',(#1352),#964,.F.);
#7004=ADVANCED_FACE('',(#1353),#965,.F.);
#7005=ADVANCED_FACE('',(#1354),#966,.F.);
#7006=ADVANCED_FACE('',(#1355),#967,.F.);
#7007=ADVANCED_FACE('',(#1356,#846),#968,.T.);
#7008=ADVANCED_FACE('',(#1357),#969,.T.);
#7009=ADVANCED_FACE('',(#1358),#757,.T.);
#7010=ADVANCED_FACE('',(#1359),#6625,.T.);
#7011=ADVANCED_FACE('',(#1360),#758,.T.);
#7012=ADVANCED_FACE('',(#1361,#847),#970,.T.);
#7033=CLOSED_SHELL('',(#6986,#6987,#6988,#6989,#6990,#6991,#6992,#6993,
#6994,#6995,#6996,#6997,#6998,#6999,#7000,#7001,#7002,#7003,#7004,#7005,
#7006,#7007,#7008,#7009,#7010,#7011,#7012));
#7755=AXIS2_PLACEMENT_3D('',#22087,#9256,#9257);
#7756=AXIS2_PLACEMENT_3D('',#22088,#9258,#9259);
#7757=AXIS2_PLACEMENT_3D('',#22104,#9261,#9262);
#7758=AXIS2_PLACEMENT_3D('',#22112,#9263,#9264);
#7759=AXIS2_PLACEMENT_3D('',#22160,#9266,#9267);
#7760=AXIS2_PLACEMENT_3D('',#22214,#9269,#9270);
#7761=AXIS2_PLACEMENT_3D('',#22262,#9272,#9273);
#7762=AXIS2_PLACEMENT_3D('',#22313,#9275,#9276);
#7763=AXIS2_PLACEMENT_3D('',#22329,#9278,#9279);
#7764=AXIS2_PLACEMENT_3D('',#22339,#9280,#9281);
#7765=AXIS2_PLACEMENT_3D('',#22363,#9283,#9284);
#7766=AXIS2_PLACEMENT_3D('',#22388,#9286,#9287);
#7767=AXIS2_PLACEMENT_3D('',#22413,#9289,#9290);
#7768=AXIS2_PLACEMENT_3D('',#22501,#9291,#9292);
#7769=AXIS2_PLACEMENT_3D('',#22503,#9293,#9294);
#7770=AXIS2_PLACEMENT_3D('',#22843,#9295,#9296);
#7771=AXIS2_PLACEMENT_3D('',#22845,#9297,#9298);
#7772=AXIS2_PLACEMENT_3D('',#22846,#9299,#9300);
#7773=AXIS2_PLACEMENT_3D('',#22939,#9301,#9302);
#7774=AXIS2_PLACEMENT_3D('',#22940,#9303,#9304);
#7775=AXIS2_PLACEMENT_3D('',#23096,#9305,#9306);
#7776=AXIS2_PLACEMENT_3D('',#23100,#9308,#9309);
#7777=AXIS2_PLACEMENT_3D('',#23101,#9310,#9311);
#7778=AXIS2_PLACEMENT_3D('',#23110,#9316,#9317);
#7779=AXIS2_PLACEMENT_3D('',#23116,#9321,#9322);
#7780=AXIS2_PLACEMENT_3D('',#23122,#9326,#9327);
#7781=AXIS2_PLACEMENT_3D('',#23128,#9331,#9332);
#7782=AXIS2_PLACEMENT_3D('',#23134,#9336,#9337);
#7783=AXIS2_PLACEMENT_3D('',#23137,#9340,#9341);
#7784=AXIS2_PLACEMENT_3D('',#23138,#9342,#9343);
#7785=AXIS2_PLACEMENT_3D('',#23140,#9344,#9345);
#7786=AXIS2_PLACEMENT_3D('',#23141,#9346,#9347);
#7787=AXIS2_PLACEMENT_3D('',#23143,#9349,#9350);
#7788=AXIS2_PLACEMENT_3D('',#23144,#9351,#9352);
#7789=AXIS2_PLACEMENT_3D('',#23145,#9353,#9354);
#7790=AXIS2_PLACEMENT_3D('',#23147,#9355,#9356);
#7791=AXIS2_PLACEMENT_3D('',#23149,#9358,#9359);
#9256=DIRECTION('axis',(0.,0.,1.));
#9257=DIRECTION('refdir',(1.,0.,0.));
#9258=DIRECTION('center_axis',(1.,0.,0.));
#9259=DIRECTION('ref_axis',(0.,1.,0.));
#9260=DIRECTION('',(-1.,0.,0.));
#9261=DIRECTION('center_axis',(1.,0.,0.));
#9262=DIRECTION('ref_axis',(0.,1.,0.));
#9263=DIRECTION('center_axis',(1.,0.,0.));
#9264=DIRECTION('ref_axis',(0.,1.,0.));
#9265=DIRECTION('',(-1.,0.,0.));
#9266=DIRECTION('center_axis',(1.,0.,0.));
#9267=DIRECTION('ref_axis',(0.,1.,0.));
#9268=DIRECTION('',(-1.,0.,0.));
#9269=DIRECTION('center_axis',(1.,0.,0.));
#9270=DIRECTION('ref_axis',(0.,1.,0.));
#9271=DIRECTION('',(-1.,0.,0.));
#9272=DIRECTION('center_axis',(1.,0.,0.));
#9273=DIRECTION('ref_axis',(0.,1.,0.));
#9274=DIRECTION('',(-1.,0.,0.));
#9275=DIRECTION('center_axis',(1.,0.,0.));
#9276=DIRECTION('ref_axis',(0.,1.,4.77055255383026E-15));
#9277=DIRECTION('',(1.,0.,0.));
#9278=DIRECTION('center_axis',(1.,0.,0.));
#9279=DIRECTION('ref_axis',(0.,1.,4.77055255383026E-15));
#9280=DIRECTION('center_axis',(1.,0.,0.));
#9281=DIRECTION('ref_axis',(0.,1.,4.77055255383026E-15));
#9282=DIRECTION('',(1.,0.,0.));
#9283=DIRECTION('center_axis',(1.,0.,0.));
#9284=DIRECTION('ref_axis',(0.,1.,4.77055255383026E-15));
#9285=DIRECTION('',(1.,0.,0.));
#9286=DIRECTION('center_axis',(1.,0.,0.));
#9287=DIRECTION('ref_axis',(0.,1.,4.77055255383026E-15));
#9288=DIRECTION('',(1.,0.,0.));
#9289=DIRECTION('center_axis',(1.,0.,0.));
#9290=DIRECTION('ref_axis',(0.,0.,-1.));
#9291=DIRECTION('center_axis',(-1.,0.,0.));
#9292=DIRECTION('ref_axis',(0.,1.,0.));
#9293=DIRECTION('center_axis',(-1.,0.,0.));
#9294=DIRECTION('ref_axis',(0.,1.,0.));
#9295=DIRECTION('center_axis',(1.,0.,0.));
#9296=DIRECTION('ref_axis',(0.,0.,-1.));
#9297=DIRECTION('center_axis',(1.,0.,0.));
#9298=DIRECTION('ref_axis',(0.,1.,0.));
#9299=DIRECTION('center_axis',(1.,0.,0.));
#9300=DIRECTION('ref_axis',(0.,1.,0.));
#9301=DIRECTION('center_axis',(-1.,0.,0.));
#9302=DIRECTION('ref_axis',(0.,1.,4.77055255383026E-15));
#9303=DIRECTION('center_axis',(1.,0.,0.));
#9304=DIRECTION('ref_axis',(0.,0.889087843978286,0.457736611699396));
#9305=DIRECTION('center_axis',(1.,0.,0.));
#9306=DIRECTION('ref_axis',(0.,1.,0.));
#9307=DIRECTION('',(0.520759202022183,-0.853703609872431,-1.04548539325081E-16));
#9308=DIRECTION('center_axis',(-1.,0.,0.));
#9309=DIRECTION('ref_axis',(0.,1.,0.));
#9310=DIRECTION('center_axis',(0.,-0.5,0.866025403784439));
#9311=DIRECTION('ref_axis',(0.,-0.866025403784439,-0.5));
#9312=DIRECTION('',(0.,0.866025403784439,0.5));
#9313=DIRECTION('',(1.,0.,0.));
#9314=DIRECTION('',(0.,-0.866025403784439,-0.5));
#9315=DIRECTION('',(1.,0.,0.));
#9316=DIRECTION('center_axis',(0.,0.5,0.866025403784439));
#9317=DIRECTION('ref_axis',(0.,-0.866025403784439,0.5));
#9318=DIRECTION('',(0.,0.866025403784439,-0.5));
#9319=DIRECTION('',(0.,-0.866025403784439,0.5));
#9320=DIRECTION('',(1.,0.,0.));
#9321=DIRECTION('center_axis',(0.,1.,-3.60555503696918E-16));
#9322=DIRECTION('ref_axis',(0.,3.60555503696918E-16,1.));
#9323=DIRECTION('',(0.,-3.60555503696918E-16,-1.));
#9324=DIRECTION('',(0.,3.60555503696918E-16,1.));
#9325=DIRECTION('',(1.,0.,0.));
#9326=DIRECTION('center_axis',(0.,0.5,-0.866025403784439));
#9327=DIRECTION('ref_axis',(0.,0.866025403784439,0.5));
#9328=DIRECTION('',(0.,-0.866025403784439,-0.5));
#9329=DIRECTION('',(0.,0.866025403784439,0.5));
#9330=DIRECTION('',(1.,0.,0.));
#9331=DIRECTION('center_axis',(0.,-0.5,-0.866025403784439));
#9332=DIRECTION('ref_axis',(0.,0.866025403784439,-0.5));
#9333=DIRECTION('',(0.,-0.866025403784439,0.5));
#9334=DIRECTION('',(0.,0.866025403784439,-0.5));
#9335=DIRECTION('',(1.,0.,0.));
#9336=DIRECTION('center_axis',(0.,-1.,-1.20185167898973E-16));
#9337=DIRECTION('ref_axis',(0.,1.20185167898973E-16,-1.));
#9338=DIRECTION('',(0.,-1.20185167898973E-16,1.));
#9339=DIRECTION('',(0.,1.20185167898973E-16,-1.));
#9340=DIRECTION('center_axis',(1.,0.,0.));
#9341=DIRECTION('ref_axis',(0.,0.,-1.));
#9342=DIRECTION('center_axis',(-1.,0.,0.));
#9343=DIRECTION('ref_axis',(0.,0.,1.));
#9344=DIRECTION('center_axis',(1.,0.,0.));
#9345=DIRECTION('ref_axis',(0.,0.,-1.));
#9346=DIRECTION('center_axis',(1.,0.,0.));
#9347=DIRECTION('ref_axis',(0.,1.,0.));
#9348=DIRECTION('',(-0.66896473162245,0.743294146247166,9.10272797026557E-17));
#9349=DIRECTION('center_axis',(1.,0.,0.));
#9350=DIRECTION('ref_axis',(0.,-0.163995302605342,-0.986461119722101));
#9351=DIRECTION('center_axis',(-1.,0.,0.));
#9352=DIRECTION('ref_axis',(0.,1.,0.));
#9353=DIRECTION('center_axis',(-1.,0.,0.));
#9354=DIRECTION('ref_axis',(0.,1.,0.));
#9355=DIRECTION('center_axis',(1.,0.,0.));
#9356=DIRECTION('ref_axis',(0.,0.,-1.));
#9357=DIRECTION('',(-0.707106781186548,-0.707106781186547,-8.65956056235493E-17));
#9358=DIRECTION('center_axis',(1.,0.,0.));
#9359=DIRECTION('ref_axis',(0.,0.,-1.));
#22087=CARTESIAN_POINT('',(0.,0.,0.));
#22088=CARTESIAN_POINT('Origin',(2.025,0.,0.));
#22089=CARTESIAN_POINT('',(0.634469692124231,-1.95442077682041,0.00165102877781057));
#22090=CARTESIAN_POINT('',(0.53273030787577,-1.95523081632926,0.00202491348536037));
#22091=CARTESIAN_POINT('',(2.025,-1.954,-2.39295984553393E-16));
#22092=CARTESIAN_POINT('',(0.408600000000001,0.862482803259043,1.75460523117329));
#22093=CARTESIAN_POINT('Ctrl Pts',(0.634469692124231,-1.95442077682041,
0.00165102877781057));
#22094=CARTESIAN_POINT('Ctrl Pts',(0.626966520753468,-1.95553671624047,
0.133139557122026));
#22095=CARTESIAN_POINT('Ctrl Pts',(0.619463349382705,-1.94333788513784,
0.26441413153127));
#22096=CARTESIAN_POINT('Ctrl Pts',(0.611960178011943,-1.91704116468773,
0.392788375779545));
#22097=CARTESIAN_POINT('Ctrl Pts',(0.575840656321609,-1.7904513644889,1.01076923620262));
#22098=CARTESIAN_POINT('Ctrl Pts',(0.539721134631274,-1.337162156549,1.561538890573));
#22099=CARTESIAN_POINT('Ctrl Pts',(0.503601612940941,-0.75508611564872,
1.80514346557071));
#22100=CARTESIAN_POINT('Ctrl Pts',(0.471934408627294,-0.244760395632316,
2.01871982226583));
#22101=CARTESIAN_POINT('Ctrl Pts',(0.440267204313647,0.364558881626702,
1.99619002455956));
#22102=CARTESIAN_POINT('Ctrl Pts',(0.408600000000001,0.863439746847564,
1.75538915071904));
#22103=CARTESIAN_POINT('',(0.408600000000001,-0.861525859670526,1.75382131162754));
#22104=CARTESIAN_POINT('Origin',(0.408600000000001,0.,0.));
#22105=CARTESIAN_POINT('Ctrl Pts',(0.408600000000001,-0.861525859670528,
1.75382131162754));
#22106=CARTESIAN_POINT('Ctrl Pts',(0.444719521690335,-1.43012887970028,
1.47450767665535));
#22107=CARTESIAN_POINT('Ctrl Pts',(0.480839043380669,-1.84834511638748,
0.900224305747275));
#22108=CARTESIAN_POINT('Ctrl Pts',(0.516958565071003,-1.9370954607764,0.276569295008137));
#22109=CARTESIAN_POINT('Ctrl Pts',(0.522215812672592,-1.95001319925531,
0.18579542381635));
#22110=CARTESIAN_POINT('Ctrl Pts',(0.527473060274181,-1.95595113187234,
0.0939756038050989));
#22111=CARTESIAN_POINT('Ctrl Pts',(0.53273030787577,-1.95523081632926,0.00202491348536037));
#22112=CARTESIAN_POINT('Origin',(2.025,0.,0.));
#22113=CARTESIAN_POINT('',(1.33446969212423,-1.9523906058954,-0.00132468018748402));
#22114=CARTESIAN_POINT('',(1.23273030787577,-1.95165222738269,-0.000920442742864252));
#22115=CARTESIAN_POINT('',(2.025,-1.954,-2.39295984553393E-16));
#22116=CARTESIAN_POINT('Ctrl Pts',(1.33446969212423,-1.9523906058954,-0.00132468018748402));
#22117=CARTESIAN_POINT('Ctrl Pts',(1.31035031756214,-1.94957125408737,0.422486472286078));
#22118=CARTESIAN_POINT('Ctrl Pts',(1.28623094300005,-1.81322651205539,0.847951210739301));
#22119=CARTESIAN_POINT('Ctrl Pts',(1.26211156843795,-1.55843747807863,1.18346739203252));
#22120=CARTESIAN_POINT('Ctrl Pts',(1.22599204674762,-1.1768828894432,1.685913421737));
#22121=CARTESIAN_POINT('Ctrl Pts',(1.18987252505729,-0.529705083115927,
1.98664078026466));
#22122=CARTESIAN_POINT('Ctrl Pts',(1.15375300336695,0.100367612944418,1.95428499231951));
#22123=CARTESIAN_POINT('Ctrl Pts',(1.11763348167662,0.730440309004762,1.92192920437435));
#22124=CARTESIAN_POINT('Ctrl Pts',(1.08151395998628,1.34340789479817,1.55649026995639));
#22125=CARTESIAN_POINT('Ctrl Pts',(1.04539443829595,1.6714805104491,1.01759080735173));
#22126=CARTESIAN_POINT('Ctrl Pts',(1.00927491660562,1.99955312610003,0.478691344747064));
#22127=CARTESIAN_POINT('Ctrl Pts',(0.973155394915283,2.04273077160847,-0.233668646044295));
#22128=CARTESIAN_POINT('Ctrl Pts',(0.937035873224949,1.78215915473901,-0.808233567143524));
#22129=CARTESIAN_POINT('Ctrl Pts',(0.900916351534615,1.52158753786956,-1.38279848824275));
#22130=CARTESIAN_POINT('Ctrl Pts',(0.864796829844281,0.957266658622202,
-1.81956833964985));
#22131=CARTESIAN_POINT('Ctrl Pts',(0.828677308153947,0.33571329746904,-1.92782633644309));
#22132=CARTESIAN_POINT('Ctrl Pts',(0.792557786463613,-0.285840063684128,
-2.03608433323634));
#22133=CARTESIAN_POINT('Ctrl Pts',(0.756438264773278,-0.964625906743106,
-1.81583047541573));
#22134=CARTESIAN_POINT('Ctrl Pts',(0.720318743082944,-1.40407363204372,
-1.36310751326752));
#22135=CARTESIAN_POINT('Ctrl Pts',(0.691702392763373,-1.75223411329688,
-1.00442948331969));
#22136=CARTESIAN_POINT('Ctrl Pts',(0.663086042443802,-1.95016469471835,
-0.499833157597696));
#22137=CARTESIAN_POINT('Ctrl Pts',(0.634469692124231,-1.95442077682041,
0.00165102877781057));
#22138=CARTESIAN_POINT('Ctrl Pts',(0.53273030787577,-1.95523081632926,0.00202491348536037));
#22139=CARTESIAN_POINT('Ctrl Pts',(0.563592581964515,-1.95100225845912,
-0.537764653671288));
#22140=CARTESIAN_POINT('Ctrl Pts',(0.59445485605326,-1.71731794149376,-1.08206425789097));
#22141=CARTESIAN_POINT('Ctrl Pts',(0.625317130142005,-1.31923087498139,
-1.44574814791387));
#22142=CARTESIAN_POINT('Ctrl Pts',(0.661436651832339,-0.853331492706804,
-1.87138392952654));
#22143=CARTESIAN_POINT('Ctrl Pts',(0.697556173522673,-0.162248276066999,
-2.04962884218167));
#22144=CARTESIAN_POINT('Ctrl Pts',(0.733675695213007,0.451679724322199,
-1.9038608795556));
#22145=CARTESIAN_POINT('Ctrl Pts',(0.769795216903341,1.0656077247114,-1.75809291692952));
#22146=CARTESIAN_POINT('Ctrl Pts',(0.805914738593676,1.60238050884999,-1.28831207902223));
#22147=CARTESIAN_POINT('Ctrl Pts',(0.842034260284009,1.8277202876157,-0.699119771386502));
#22148=CARTESIAN_POINT('Ctrl Pts',(0.878153781974343,2.0530600663814,-0.109927463750781));
#22149=CARTESIAN_POINT('Ctrl Pts',(0.914273303664676,1.96696683977422,0.598676313613372));
#22150=CARTESIAN_POINT('Ctrl Pts',(0.95039282535501,1.60693687797777,1.11679866753813));
#22151=CARTESIAN_POINT('Ctrl Pts',(0.986512347045345,1.24690691618132,1.63492102146289));
#22152=CARTESIAN_POINT('Ctrl Pts',(1.02263186873568,0.612940219195604,1.96256195194826));
#22153=CARTESIAN_POINT('Ctrl Pts',(1.05875139042601,-0.0179439077178916,
1.95675679282911));
#22154=CARTESIAN_POINT('Ctrl Pts',(1.09487091211635,-0.648828034631387,
1.95095163370997));
#22155=CARTESIAN_POINT('Ctrl Pts',(1.13099043380668,-1.27662959147266,1.61170038498632));
#22156=CARTESIAN_POINT('Ctrl Pts',(1.16710995549701,-1.62711418555438,1.08712141076958));
#22157=CARTESIAN_POINT('Ctrl Pts',(1.18898340628993,-1.83936249792265,0.769444103802367));
#22158=CARTESIAN_POINT('Ctrl Pts',(1.21085685708285,-1.94990937996376,0.383800904758547));
#22159=CARTESIAN_POINT('Ctrl Pts',(1.23273030787577,-1.95165222738269,-0.000920442742864252));
#22160=CARTESIAN_POINT('Origin',(2.025,0.,0.));
#22161=CARTESIAN_POINT('',(2.03446969212423,-1.95576993562625,0.00117566504278285));
#22162=CARTESIAN_POINT('',(1.93273030787577,-1.95653837240827,0.000668140733460532));
#22163=CARTESIAN_POINT('',(2.025,-1.954,-2.39295984553393E-16));
#22164=CARTESIAN_POINT('Ctrl Pts',(2.03446969212423,-1.95576993562625,0.00117566504278285));
#22165=CARTESIAN_POINT('Ctrl Pts',(2.02985363606114,-1.95635392431848,0.0819247817601888));
#22166=CARTESIAN_POINT('Ctrl Pts',(2.02523757999806,-1.95176291393843,0.162607088786322));
#22167=CARTESIAN_POINT('Ctrl Pts',(2.02062152393497,-1.94176643790063,0.242614011988077));
#22168=CARTESIAN_POINT('Ctrl Pts',(1.98450200224464,-1.86354643187397,0.868648825791863));
#22169=CARTESIAN_POINT('Ctrl Pts',(1.9483824805543,-1.45436685550396,1.45333202356739));
#22170=CARTESIAN_POINT('Ctrl Pts',(1.91226295886397,-0.892984570149823,
1.74123449713021));
#22171=CARTESIAN_POINT('Ctrl Pts',(1.87614343717363,-0.331602284795679,
2.02913697069302));
#22172=CARTESIAN_POINT('Ctrl Pts',(1.8400239154833,0.381982709542597,2.02025872004313));
#22173=CARTESIAN_POINT('Ctrl Pts',(1.80390439379297,0.936028534854556,1.71847869934669));
#22174=CARTESIAN_POINT('Ctrl Pts',(1.76778487210263,1.49007436016651,1.41669867865025));
#22175=CARTESIAN_POINT('Ctrl Pts',(1.73166535041229,1.88458101645215,0.822016887907262));
#22176=CARTESIAN_POINT('Ctrl Pts',(1.69554582872196,1.94720150826564,0.194229666915167));
#22177=CARTESIAN_POINT('Ctrl Pts',(1.65942630703163,2.00982200007913,-0.433557554076929));
#22178=CARTESIAN_POINT('Ctrl Pts',(1.6233067853413,1.74055632742047,-1.09445020531813));
#22179=CARTESIAN_POINT('Ctrl Pts',(1.58718726365096,1.25703793962356,-1.49972501984526));
#22180=CARTESIAN_POINT('Ctrl Pts',(1.55106774196063,0.773519551826663,-1.90499983437239));
#22181=CARTESIAN_POINT('Ctrl Pts',(1.51494822027029,0.0757484488915239,
-2.05465681218543));
#22182=CARTESIAN_POINT('Ctrl Pts',(1.47882869857996,-0.531442461668977,
-1.88331767599797));
#22183=CARTESIAN_POINT('Ctrl Pts',(1.44270917688962,-1.13863337222948,-1.7119785398105));
#22184=CARTESIAN_POINT('Ctrl Pts',(1.40658965519929,-1.65524409041534,-1.21964328962253));
#22185=CARTESIAN_POINT('Ctrl Pts',(1.37047013350896,-1.85558376403649,-0.621393314087894));
#22186=CARTESIAN_POINT('Ctrl Pts',(1.35846998638071,-1.92214349258685,-0.422634100512704));
#22187=CARTESIAN_POINT('Ctrl Pts',(1.34646983925247,-1.95379332205687,-0.212184052646743));
#22188=CARTESIAN_POINT('Ctrl Pts',(1.33446969212423,-1.9523906058954,-0.00132468018748402));
#22189=CARTESIAN_POINT('Ctrl Pts',(1.23273030787577,-1.95165222738269,-0.000920442742864252));
#22190=CARTESIAN_POINT('Ctrl Pts',(1.24697637877319,-1.95278733533289,-0.251487563776593));
#22191=CARTESIAN_POINT('Ctrl Pts',(1.2612224496706,-1.90776937317109,-0.501663648953817));
#22192=CARTESIAN_POINT('Ctrl Pts',(1.27546852056802,-1.81463610591833,-0.732417095986825));
#22193=CARTESIAN_POINT('Ctrl Pts',(1.31158804225835,-1.57850580087837,-1.31746992881668));
#22194=CARTESIAN_POINT('Ctrl Pts',(1.34770756394868,-1.03307755947628,-1.77766889476657));
#22195=CARTESIAN_POINT('Ctrl Pts',(1.38382708563902,-0.416639625931859,
-1.91199265209425));
#22196=CARTESIAN_POINT('Ctrl Pts',(1.41994660732935,0.199798307612564,-2.04631640942193));
#22197=CARTESIAN_POINT('Ctrl Pts',(1.45606612901969,0.887245933299322,-1.85476495812738));
#22198=CARTESIAN_POINT('Ctrl Pts',(1.49218565071002,1.34538450854715,-1.42100803903579));
#22199=CARTESIAN_POINT('Ctrl Pts',(1.52830517240036,1.80352308379497,-0.987251119944189));
#22200=CARTESIAN_POINT('Ctrl Pts',(1.56442469409069,2.03235260860386,-0.311288733055544));
#22201=CARTESIAN_POINT('Ctrl Pts',(1.60054421578102,1.93190264788241,0.311566717611194));
#22202=CARTESIAN_POINT('Ctrl Pts',(1.63666373747136,1.83145268716095,0.934422168277935));
#22203=CARTESIAN_POINT('Ctrl Pts',(1.67278325916169,1.40172324090913,1.50417068272276));
#22204=CARTESIAN_POINT('Ctrl Pts',(1.70890278085203,0.830450180305799,1.77191139223846));
#22205=CARTESIAN_POINT('Ctrl Pts',(1.74502230254236,0.259177119702472,2.03965210175416));
#22206=CARTESIAN_POINT('Ctrl Pts',(1.78114182423269,-0.453639555252363,
2.00538500634072));
#22207=CARTESIAN_POINT('Ctrl Pts',(1.81726134592303,-0.996594329999513,
1.68407843139874));
#22208=CARTESIAN_POINT('Ctrl Pts',(1.85338086761336,-1.53954910474667,1.36277185645676));
#22209=CARTESIAN_POINT('Ctrl Pts',(1.8895003893037,-1.91264197928614,0.754425801986236));
#22210=CARTESIAN_POINT('Ctrl Pts',(1.92561991099403,-1.95288065385836,0.124807613218624));
#22211=CARTESIAN_POINT('Ctrl Pts',(1.92799004328794,-1.95552108146107,0.0834926031576606));
#22212=CARTESIAN_POINT('Ctrl Pts',(1.93036017558186,-1.95672828122377,0.0420859979926118));
#22213=CARTESIAN_POINT('Ctrl Pts',(1.93273030787577,-1.95653837240827,0.000668140733460532));
#22214=CARTESIAN_POINT('Origin',(2.025,0.,0.));
#22215=CARTESIAN_POINT('',(2.73446969212423,-1.95150456667077,-0.000783624415817835));
#22216=CARTESIAN_POINT('',(2.63273030787577,-1.95117066719132,-0.000238996725395994));
#22217=CARTESIAN_POINT('',(2.025,-1.954,-2.39295984553393E-16));
#22218=CARTESIAN_POINT('Ctrl Pts',(2.73446969212423,-1.95150456667077,-0.000783624415817835));
#22219=CARTESIAN_POINT('Ctrl Pts',(2.71323743286981,-1.9500751429531,0.372726459605641));
#22220=CARTESIAN_POINT('Ctrl Pts',(2.6920051736154,-1.84631774470697,0.746969407126199));
#22221=CARTESIAN_POINT('Ctrl Pts',(2.67077291436098,-1.64564170315827,1.05885167694053));
#22222=CARTESIAN_POINT('Ctrl Pts',(2.63465339267065,-1.30425916121605,1.58941407609013));
#22223=CARTESIAN_POINT('Ctrl Pts',(2.59853387098031,-0.682398562187567,
1.93950756724007));
#22224=CARTESIAN_POINT('Ctrl Pts',(2.56241434928998,-0.0517180701627423,
1.95618191441976));
#22225=CARTESIAN_POINT('Ctrl Pts',(2.52629482759964,0.578962421862082,1.97285626159946));
#22226=CARTESIAN_POINT('Ctrl Pts',(2.49017530590931,1.21846280688325,1.65611146480892));
#22227=CARTESIAN_POINT('Ctrl Pts',(2.45405578421898,1.58740000205626,1.14432599796594));
#22228=CARTESIAN_POINT('Ctrl Pts',(2.41793626252864,1.95633719722927,0.63254053112295));
#22229=CARTESIAN_POINT('Ctrl Pts',(2.38181674083831,2.05471120255412,-0.0742856057724776));
#22230=CARTESIAN_POINT('Ctrl Pts',(2.34569721914798,1.83954900887748,-0.667364969659822));
#22231=CARTESIAN_POINT('Ctrl Pts',(2.30957769745764,1.62438681520084,-1.26044433354716));
#22232=CARTESIAN_POINT('Ctrl Pts',(2.27345817576731,1.0956884225227,-1.73977692442642));
#22233=CARTESIAN_POINT('Ctrl Pts',(2.23733865407697,0.484423001993893,-1.8959572442284));
#22234=CARTESIAN_POINT('Ctrl Pts',(2.20121913238664,-0.126842418534916,
-2.05213756403038));
#22235=CARTESIAN_POINT('Ctrl Pts',(2.1650996106963,-0.820674866914401,-1.88516561275509));
#22236=CARTESIAN_POINT('Ctrl Pts',(2.12898008900597,-1.29396087326249,-1.46798642220142));
#22237=CARTESIAN_POINT('Ctrl Pts',(2.09747662337872,-1.70676117445901,-1.10412251495796));
#22238=CARTESIAN_POINT('Ctrl Pts',(2.06597315775148,-1.95178435411669,-0.549917516705958));
#22239=CARTESIAN_POINT('Ctrl Pts',(2.03446969212423,-1.95576993562625,0.00117566504278285));
#22240=CARTESIAN_POINT('Ctrl Pts',(1.93273030787577,-1.95653837240827,0.000668140733460532));
#22241=CARTESIAN_POINT('Ctrl Pts',(1.96647969727219,-1.95383417459587,-0.589099525904457));
#22242=CARTESIAN_POINT('Ctrl Pts',(2.00022908666861,-1.66784938341305,-1.18114869016093));
#22243=CARTESIAN_POINT('Ctrl Pts',(2.03397847606503,-1.20286828249105,-1.54351134325543));
#22244=CARTESIAN_POINT('Ctrl Pts',(2.07009799775536,-0.705232761946527,
-1.93132178789718));
#22245=CARTESIAN_POINT('Ctrl Pts',(2.1062175194457,-0.002577246252485,-2.05605235411599));
#22246=CARTESIAN_POINT('Ctrl Pts',(2.14233704113603,0.598131172672099,-1.86321201845565));
#22247=CARTESIAN_POINT('Ctrl Pts',(2.17845656282637,1.19883959159669,-1.67037168279531));
#22248=CARTESIAN_POINT('Ctrl Pts',(2.2145760845167,1.69760091375181,-1.15996044525583));
#22249=CARTESIAN_POINT('Ctrl Pts',(2.25069560620703,1.87652291444005,-0.554960470090062));
#22250=CARTESIAN_POINT('Ctrl Pts',(2.28681512789737,2.05544491512828,0.0500395050757017));
#22251=CARTESIAN_POINT('Ctrl Pts',(2.3229346495877,1.91452759434962,0.749628217867738));
#22252=CARTESIAN_POINT('Ctrl Pts',(2.35905417127804,1.51533268176147,1.23817876420054));
#22253=CARTESIAN_POINT('Ctrl Pts',(2.39517369296837,1.11613776917333,1.72672931053334));
#22254=CARTESIAN_POINT('Ctrl Pts',(2.43129321465871,0.458665264775706,2.0042416904069));
#22255=CARTESIAN_POINT('Ctrl Pts',(2.46741273634904,-0.169855919296459,
1.94947926082059));
#22256=CARTESIAN_POINT('Ctrl Pts',(2.50353225803937,-0.798377103368625,
1.89471683123428));
#22257=CARTESIAN_POINT('Ctrl Pts',(2.53965177972971,-1.39794696711534,1.50767959218809));
#22258=CARTESIAN_POINT('Ctrl Pts',(2.57577130142004,-1.7066347542496,0.957452505089308));
#22259=CARTESIAN_POINT('Ctrl Pts',(2.59475763690528,-1.86889742032186,0.668223977693796));
#22260=CARTESIAN_POINT('Ctrl Pts',(2.61374397239053,-1.95078614203936,0.333904285110699));
#22261=CARTESIAN_POINT('Ctrl Pts',(2.63273030787577,-1.95117066719132,-0.000238996725395994));
#22262=CARTESIAN_POINT('Origin',(2.025,0.,0.));
#22263=CARTESIAN_POINT('',(3.43446969212423,-1.95694215816793,0.000613609334558611));
#22264=CARTESIAN_POINT('',(3.33273030787577,-1.95689202958038,-0.000120183693368507));
#22265=CARTESIAN_POINT('',(2.025,-1.954,-2.39295984553393E-16));
#22266=CARTESIAN_POINT('Ctrl Pts',(3.43446969212423,-1.95694215816793,0.000613609334558611));
#22267=CARTESIAN_POINT('Ctrl Pts',(3.43274075136882,-1.95706861247031,0.0308306145688404));
#22268=CARTESIAN_POINT('Ctrl Pts',(3.43101181061341,-1.95644434477529,0.0610420651850611));
#22269=CARTESIAN_POINT('Ctrl Pts',(3.42928286985799,-1.95505445535266,0.0912168450879343));
#22270=CARTESIAN_POINT('Ctrl Pts',(3.39316334816766,-1.92601809827063,0.721602018085349));
#22271=CARTESIAN_POINT('Ctrl Pts',(3.35704382647733,-1.56283440190639,1.33598265404732));
#22272=CARTESIAN_POINT('Ctrl Pts',(3.32092430478699,-1.02535127629691,1.66653914851539));
#22273=CARTESIAN_POINT('Ctrl Pts',(3.28480478309666,-0.48786815068743,1.99709564298347));
#22274=CARTESIAN_POINT('Ctrl Pts',(3.24868526140633,0.223914404167301,2.04382799595763));
#22275=CARTESIAN_POINT('Ctrl Pts',(3.21256573971599,0.799644251583046,1.78602872489919));
#22276=CARTESIAN_POINT('Ctrl Pts',(3.17644621802565,1.3753740989988,1.52822945384073));
#22277=CARTESIAN_POINT('Ctrl Pts',(3.14032669633532,1.81505123897556,0.965898558749655));
#22278=CARTESIAN_POINT('Ctrl Pts',(3.10420717464499,1.92628208012454,0.344850989150182));
#22279=CARTESIAN_POINT('Ctrl Pts',(3.06808765295465,2.03751292127353,-0.276196580449285));
#22280=CARTESIAN_POINT('Ctrl Pts',(3.03196813126432,1.82029746359473,-0.955960824557148));
#22281=CARTESIAN_POINT('Ctrl Pts',(2.99584860957399,1.36969361078797,-1.39755401117372));
#22282=CARTESIAN_POINT('Ctrl Pts',(2.95972908788365,0.919089757981196,-1.83914719779029));
#22283=CARTESIAN_POINT('Ctrl Pts',(2.92360956619332,0.235097510046449,-2.04256932691557));
#22284=CARTESIAN_POINT('Ctrl Pts',(2.88749004450298,-0.383555026741606,
-1.91891070488933));
#22285=CARTESIAN_POINT('Ctrl Pts',(2.85137052281265,-1.00220756352966,-1.79525208286309));
#22286=CARTESIAN_POINT('Ctrl Pts',(2.81525100112232,-1.55552038917102,-1.34451270968533));
#22287=CARTESIAN_POINT('Ctrl Pts',(2.77913147943199,-1.80172455956373,-0.763627369521821));
#22288=CARTESIAN_POINT('Ctrl Pts',(2.76424421699607,-1.90320170892571,-0.524205801918239));
#22289=CARTESIAN_POINT('Ctrl Pts',(2.74935695456015,-1.9525068248743,-0.262674861549822));
#22290=CARTESIAN_POINT('Ctrl Pts',(2.73446969212423,-1.95150456667077,-0.000783624415817835));
#22291=CARTESIAN_POINT('Ctrl Pts',(2.63273030787577,-1.95117066719132,-0.000238996725395994));
#22292=CARTESIAN_POINT('Ctrl Pts',(2.64986349408086,-1.95151766100874,-0.301768434637608));
#22293=CARTESIAN_POINT('Ctrl Pts',(2.66699668028595,-1.88549433057532,-0.603154218124976));
#22294=CARTESIAN_POINT('Ctrl Pts',(2.68412986649104,-1.75227012486661,-0.871132062271862));
#22295=CARTESIAN_POINT('Ctrl Pts',(2.72024938818138,-1.47141199782754,-1.43607260738287));
#22296=CARTESIAN_POINT('Ctrl Pts',(2.75636890987171,-0.89189003322759,-1.85253676245349));
#22297=CARTESIAN_POINT('Ctrl Pts',(2.79248843156204,-0.266884103330787,
-1.93858097541276));
#22298=CARTESIAN_POINT('Ctrl Pts',(2.82860795325238,0.358121826566009,-2.02462518837203));
#22299=CARTESIAN_POINT('Ctrl Pts',(2.86472747494271,1.02861172175966,-1.78024945921995));
#22300=CARTESIAN_POINT('Ctrl Pts',(2.90084699663305,1.45168171419148,-1.31222127716369));
#22301=CARTESIAN_POINT('Ctrl Pts',(2.93696651832338,1.87475170662331,-0.844193095107442));
#22302=CARTESIAN_POINT('Ctrl Pts',(2.97308604001372,2.0504017962933,-0.152512460147026));
#22303=CARTESIAN_POINT('Ctrl Pts',(3.00920556170405,1.90187502389171,0.460662992754071));
#22304=CARTESIAN_POINT('Ctrl Pts',(3.04532508339438,1.75334825149011,1.07383844565517));
#22305=CARTESIAN_POINT('Ctrl Pts',(3.08144460508472,1.28064461701691,1.60850871649694));
#22306=CARTESIAN_POINT('Ctrl Pts',(3.11756412677505,0.690313345419868,1.83106554216969));
#22307=CARTESIAN_POINT('Ctrl Pts',(3.15368364846538,0.099982073822824,2.05362236784244));
#22308=CARTESIAN_POINT('Ctrl Pts',(3.18980317015572,-0.607976834898069,
1.96406574834616));
#22309=CARTESIAN_POINT('Ctrl Pts',(3.22592269184605,-1.12435700524545,1.60157436757165));
#22310=CARTESIAN_POINT('Ctrl Pts',(3.26152523052262,-1.63334616474276,1.24427136908255));
#22311=CARTESIAN_POINT('Ctrl Pts',(3.2971277691992,-1.95620151659337,0.621790789891298));
#22312=CARTESIAN_POINT('Ctrl Pts',(3.33273030787577,-1.95689202958038,-0.000120183693368507));
#22313=CARTESIAN_POINT('Origin',(-0.885456225603702,0.,0.));
#22314=CARTESIAN_POINT('',(2.9645437743963,-1.55351348692753,-0.000623811555172185));
#22315=CARTESIAN_POINT('',(3.1026562256037,-1.5578012360145,-9.56321627601668E-5));
#22316=CARTESIAN_POINT('',(-0.885456225603702,-1.5555,-7.61108830709034E-15));
#22317=CARTESIAN_POINT('',(3.646,-1.53400205074397,0.257716818064529));
#22318=CARTESIAN_POINT('Ctrl Pts',(2.9645437743963,-1.55351348692753,-0.000623811555172191));
#22319=CARTESIAN_POINT('Ctrl Pts',(2.97943103683221,-1.554311343957,-0.209104783593014));
#22320=CARTESIAN_POINT('Ctrl Pts',(3.03043782095846,-1.41983356141065,-0.922420232737971));
#22321=CARTESIAN_POINT('Ctrl Pts',(3.11756412677505,-0.357346860176684,
-1.78794253319936));
#22322=CARTESIAN_POINT('Ctrl Pts',(3.22592269184605,1.2761484443205,-1.30213426013737));
#22323=CARTESIAN_POINT('Ctrl Pts',(3.33428125691706,1.79489764250785,0.32126381822974));
#22324=CARTESIAN_POINT('Ctrl Pts',(3.44263982198805,0.744870327409823,1.66421014471004));
#22325=CARTESIAN_POINT('Ctrl Pts',(3.54654606968238,-0.88514792232698,1.55719067973231));
#22326=CARTESIAN_POINT('Ctrl Pts',(3.61433279568635,-1.45984003145562,0.691579922874265));
#22327=CARTESIAN_POINT('Ctrl Pts',(3.646,-1.53590465648925,0.257207812787695));
#22328=CARTESIAN_POINT('',(3.646,-0.254962570226321,1.53446223081039));
#22329=CARTESIAN_POINT('Origin',(3.646,0.,0.));
#22330=CARTESIAN_POINT('Ctrl Pts',(3.1026562256037,-1.55780222723249,-9.5673354675919E-5));
#22331=CARTESIAN_POINT('Ctrl Pts',(3.10317320861747,-1.55781020924886,-0.00728468162261492));
#22332=CARTESIAN_POINT('Ctrl Pts',(3.13980971332156,-1.55454362905802,-0.516733977523194));
#22333=CARTESIAN_POINT('Ctrl Pts',(3.21256573971599,-1.00543213394195,-1.52103014244754));
#22334=CARTESIAN_POINT('Ctrl Pts',(3.320924304787,0.68997158388018,-1.68716896408801));
#22335=CARTESIAN_POINT('Ctrl Pts',(3.429282869858,1.78424156303041,-0.380380645529688));
#22336=CARTESIAN_POINT('Ctrl Pts',(3.53764143492899,1.31614849123568,1.26120506567147));
#22337=CARTESIAN_POINT('Ctrl Pts',(3.60988047830967,0.242522465892156,1.61712315325676));
#22338=CARTESIAN_POINT('Ctrl Pts',(3.646,-0.254962570226321,1.53446223081039));
#22339=CARTESIAN_POINT('Origin',(-0.885456225603702,0.,0.));
#22340=CARTESIAN_POINT('',(2.2645437743963,-1.55690897383144,0.000935899167884407));
#22341=CARTESIAN_POINT('',(2.4026562256037,-1.5532476831198,-0.000190255581553472));
#22342=CARTESIAN_POINT('',(-0.885456225603702,-1.5555,-7.61108830709034E-15));
#22343=CARTESIAN_POINT('Ctrl Pts',(2.2645437743963,-1.55690897383144,0.000935899167884323));
#22344=CARTESIAN_POINT('Ctrl Pts',(2.29604724002354,-1.55373621434417,-0.437766989373654));
#22345=CARTESIAN_POINT('Ctrl Pts',(2.36367022734113,-1.13505001352398,-1.38477120961871));
#22346=CARTESIAN_POINT('Ctrl Pts',(2.46741273634904,0.451357723348635,-1.76654291251687));
#22347=CARTESIAN_POINT('Ctrl Pts',(2.57577130142004,1.71398364424552,-0.621811318178061));
#22348=CARTESIAN_POINT('Ctrl Pts',(2.68412986649104,1.47904899949198,1.06621537978638));
#22349=CARTESIAN_POINT('Ctrl Pts',(2.79248843156204,-0.0481918125352924,
1.82265836557096));
#22350=CARTESIAN_POINT('Ctrl Pts',(2.88595973419713,-1.32926753649534,1.10144162772121));
#22351=CARTESIAN_POINT('Ctrl Pts',(2.94331151514188,-1.55237558078994,0.296712388903057));
#22352=CARTESIAN_POINT('Ctrl Pts',(2.9645437743963,-1.55351348692753,-0.000623811555172191));
#22353=CARTESIAN_POINT('Ctrl Pts',(2.4026562256037,-1.5532476831198,-0.000190255581553507));
#22354=CARTESIAN_POINT('Ctrl Pts',(2.4197894118088,-1.5535239107979,-0.240225588576664));
#22355=CARTESIAN_POINT('Ctrl Pts',(2.47304211970422,-1.39016363968781,-0.985938702047525));
#22356=CARTESIAN_POINT('Ctrl Pts',(2.56241434928998,-0.248663526484289,
-1.80625943050602));
#22357=CARTESIAN_POINT('Ctrl Pts',(2.67077291436098,1.35258575494928,-1.22264666689896));
#22358=CARTESIAN_POINT('Ctrl Pts',(2.77913147943198,1.77206945169698,0.429209875088153));
#22359=CARTESIAN_POINT('Ctrl Pts',(2.88749004450298,0.643168985847878,1.70609770460869));
#22360=CARTESIAN_POINT('Ctrl Pts',(2.99533162656023,-1.03949642371216,1.49324096396001));
#22361=CARTESIAN_POINT('Ctrl Pts',(3.06705368692713,-1.55725253790225,0.494982381615103));
#22362=CARTESIAN_POINT('Ctrl Pts',(3.1026562256037,-1.55780222723249,-9.5673354675919E-5));
#22363=CARTESIAN_POINT('Origin',(-0.885456225603702,0.,0.));
#22364=CARTESIAN_POINT('',(1.5645437743963,-1.55421882675041,-0.00105452406940307));
#22365=CARTESIAN_POINT('',(1.7026562256037,-1.55752069512848,0.000531879688266731));
#22366=CARTESIAN_POINT('',(-0.885456225603702,-1.5555,-7.61108830709034E-15));
#22367=CARTESIAN_POINT('Ctrl Pts',(1.5645437743963,-1.55421882675041,-0.00105452406940303));
#22368=CARTESIAN_POINT('Ctrl Pts',(1.57654392152454,-1.55533547208775,-0.168911102298873));
#22369=CARTESIAN_POINT('Ctrl Pts',(1.62466359034311,-1.45430488205528,-0.840696475689404));
#22370=CARTESIAN_POINT('Ctrl Pts',(1.70890278085203,-0.495166959245057,
-1.75476463681813));
#22371=CARTESIAN_POINT('Ctrl Pts',(1.81726134592303,1.17123470495496,-1.39735712045959));
#22372=CARTESIAN_POINT('Ctrl Pts',(1.92561991099403,1.81428908646041,0.180972233182718));
#22373=CARTESIAN_POINT('Ctrl Pts',(2.03397847606503,0.872136931108851,1.60117826005178));
#22374=CARTESIAN_POINT('Ctrl Pts',(2.14233704113603,-0.832031122156023,
1.62238110378654));
#22375=CARTESIAN_POINT('Ctrl Pts',(2.21919214057979,-1.52512187202985,0.632012719372306));
#22376=CARTESIAN_POINT('Ctrl Pts',(2.25992771833321,-1.55737386349918,0.0652169897789001));
#22377=CARTESIAN_POINT('Ctrl Pts',(2.2645437743963,-1.55690897383144,0.000935899167884323));
#22378=CARTESIAN_POINT('Ctrl Pts',(1.7026562256037,-1.55752069512848,0.000531879688266792));
#22379=CARTESIAN_POINT('Ctrl Pts',(1.73640561500012,-1.55536799313402,-0.468958194751484));
#22380=CARTESIAN_POINT('Ctrl Pts',(1.80627452608688,-1.08405821641942,-1.44466937944663));
#22381=CARTESIAN_POINT('Ctrl Pts',(1.91226295886397,0.557303862904986,-1.73603266764626));
#22382=CARTESIAN_POINT('Ctrl Pts',(2.02062152393497,1.74843472771405,-0.517079730093531));
#22383=CARTESIAN_POINT('Ctrl Pts',(2.12898008900597,1.41189906885343,1.15366271015419));
#22384=CARTESIAN_POINT('Ctrl Pts',(2.23733865407697,-0.158262365011203,
1.81641169719614));
#22385=CARTESIAN_POINT('Ctrl Pts',(2.32856403294288,-1.36373938799973,1.03824633745719));
#22386=CARTESIAN_POINT('Ctrl Pts',(2.38366989011846,-1.55294157827136,0.265807633310998));
#22387=CARTESIAN_POINT('Ctrl Pts',(2.4026562256037,-1.5532476831198,-0.000190255581553507));
#22388=CARTESIAN_POINT('Origin',(-0.885456225603702,0.,0.));
#22389=CARTESIAN_POINT('',(0.864543774396297,-1.55583496332863,0.00131431692112688));
#22390=CARTESIAN_POINT('',(1.0026562256037,-1.55363103362015,-0.000732727065787808));
#22391=CARTESIAN_POINT('',(-0.885456225603702,-1.5555,-7.61108830709034E-15));
#22392=CARTESIAN_POINT('Ctrl Pts',(0.864543774396297,-1.55583496332863,
0.00131431692112695));
#22393=CARTESIAN_POINT('Ctrl Pts',(0.893160124715868,-1.55244686931136,
-0.39789686624525));
#22394=CARTESIAN_POINT('Ctrl Pts',(0.957895996725773,-1.19600466962952,
-1.30659638604676));
#22395=CARTESIAN_POINT('Ctrl Pts',(1.05875139042601,0.312808167767432,-1.79617914851027));
#22396=CARTESIAN_POINT('Ctrl Pts',(1.16710995549701,1.66050693082158,-0.753094956293683));
#22397=CARTESIAN_POINT('Ctrl Pts',(1.27546852056802,1.55739102357227,0.948147570332657));
#22398=CARTESIAN_POINT('Ctrl Pts',(1.38382708563902,0.093515261491943,1.82088082901303));
#22399=CARTESIAN_POINT('Ctrl Pts',(1.48018550358178,-1.28089611724802,1.18222619744519));
#22400=CARTESIAN_POINT('Ctrl Pts',(1.5404243998342,-1.55197445533925,0.336324313019962));
#22401=CARTESIAN_POINT('Ctrl Pts',(1.5645437743963,-1.55421882675041,-0.00105452406940303));
#22402=CARTESIAN_POINT('Ctrl Pts',(1.0026562256037,-1.55363103362015,-0.000732727065787947));
#22403=CARTESIAN_POINT('Ctrl Pts',(1.01690229650112,-1.55453464693465,-0.200199030427076));
#22404=CARTESIAN_POINT('Ctrl Pts',(1.06726788908887,-1.42783653745201,-0.904292141434522));
#22405=CARTESIAN_POINT('Ctrl Pts',(1.15375300336695,-0.388197806685981,
-1.78147566906063));
#22406=CARTESIAN_POINT('Ctrl Pts',(1.26211156843795,1.2535495552727,-1.3240166887812));
#22407=CARTESIAN_POINT('Ctrl Pts',(1.37047013350896,1.8000352141881,0.290301877450055));
#22408=CARTESIAN_POINT('Ctrl Pts',(1.47882869857996,0.773764763351813,1.65096279999703));
#22409=CARTESIAN_POINT('Ctrl Pts',(1.58718726365096,-0.928568406390638,
1.56912687330982));
#22410=CARTESIAN_POINT('Ctrl Pts',(1.66179643932554,-1.54206571520519,0.568789711399914));
#22411=CARTESIAN_POINT('Ctrl Pts',(1.70028609330979,-1.55767187381964,0.0335029528543981));
#22412=CARTESIAN_POINT('Ctrl Pts',(1.7026562256037,-1.55752069512848,0.000531879688266792));
#22413=CARTESIAN_POINT('Origin',(3.646,2.59090492670967E-16,0.));
#22414=CARTESIAN_POINT('',(3.646,0.629287956476874,-1.84989531266857));
#22415=CARTESIAN_POINT('Ctrl Pts',(3.646,-1.53590465648925,0.257207812787684));
#22416=CARTESIAN_POINT('Ctrl Pts',(3.646,-1.55437165720027,0.196895341718919));
#22417=CARTESIAN_POINT('Ctrl Pts',(3.646,-1.56896355683948,0.135616641599751));
#22418=CARTESIAN_POINT('Ctrl Pts',(3.646,-1.5794868132962,0.0736940107076772));
#22419=CARTESIAN_POINT('Ctrl Pts',(3.646,-1.58951842709423,0.014664382282102));
#22420=CARTESIAN_POINT('Ctrl Pts',(3.646,-1.5958536213326,-0.0449514371865003));
#22421=CARTESIAN_POINT('Ctrl Pts',(3.646,-1.59865979572508,-0.104879712275592));
#22422=CARTESIAN_POINT('Ctrl Pts',(3.646,-1.59931069948911,-0.118780323702925));
#22423=CARTESIAN_POINT('Ctrl Pts',(3.646,-1.59977152479897,-0.132697823616271));
#22424=CARTESIAN_POINT('Ctrl Pts',(3.646,-1.60004398707201,-0.146628916982726));
#22425=CARTESIAN_POINT('Ctrl Pts',(3.646,-1.60029819926649,-0.159626877312327));
#22426=CARTESIAN_POINT('Ctrl Pts',(3.646,-1.60038827226624,-0.172631782210399));
#22427=CARTESIAN_POINT('Ctrl Pts',(3.646,-1.60031610868448,-0.185632728843391));
#22428=CARTESIAN_POINT('Ctrl Pts',(3.646,-1.59997115748781,-0.247778924875277));
#22429=CARTESIAN_POINT('Ctrl Pts',(3.646,-1.59592448582643,-0.309888778101361));
#22430=CARTESIAN_POINT('Ctrl Pts',(3.646,-1.58837167340201,-0.371662510966953));
#22431=CARTESIAN_POINT('Ctrl Pts',(3.646,-1.58235446873971,-0.420876654324364));
#22432=CARTESIAN_POINT('Ctrl Pts',(3.646,-1.57411085537686,-0.469878150447174));
#22433=CARTESIAN_POINT('Ctrl Pts',(3.646,-1.56371690971211,-0.518521573067589));
#22434=CARTESIAN_POINT('Ctrl Pts',(3.646,-1.55949291302958,-0.538289778752235));
#22435=CARTESIAN_POINT('Ctrl Pts',(3.646,-1.55491355506823,-0.557998881141082));
#22436=CARTESIAN_POINT('Ctrl Pts',(3.646,-1.54998301914068,-0.577639185380113));
#22437=CARTESIAN_POINT('Ctrl Pts',(3.646,-1.54698757787163,-0.589571230642318));
#22438=CARTESIAN_POINT('Ctrl Pts',(3.646,-1.54386473422877,-0.601468946211907));
#22439=CARTESIAN_POINT('Ctrl Pts',(3.646,-1.54061666379623,-0.613327738526289));
#22440=CARTESIAN_POINT('Ctrl Pts',(3.646,-1.52355820100381,-0.675608643962078));
#22441=CARTESIAN_POINT('Ctrl Pts',(3.646,-1.50304441626246,-0.736836650927299));
#22442=CARTESIAN_POINT('Ctrl Pts',(3.646,-1.47927170237122,-0.796705417992335));
#22443=CARTESIAN_POINT('Ctrl Pts',(3.646,-1.45499081172395,-0.857853968088201));
#22444=CARTESIAN_POINT('Ctrl Pts',(3.646,-1.42731013062283,-0.917585613768136));
#22445=CARTESIAN_POINT('Ctrl Pts',(3.646,-1.39638521586208,-0.975578488374583));
#22446=CARTESIAN_POINT('Ctrl Pts',(3.646,-1.3746359269342,-1.01636449523448));
#22447=CARTESIAN_POINT('Ctrl Pts',(3.646,-1.35128083281079,-1.05629059526188));
#22448=CARTESIAN_POINT('Ctrl Pts',(3.646,-1.32635893912807,-1.09524162657284));
#22449=CARTESIAN_POINT('Ctrl Pts',(3.646,-1.31177207824354,-1.11803978478166));
#22450=CARTESIAN_POINT('Ctrl Pts',(3.646,-1.29664823418257,-1.14050383295085));
#22451=CARTESIAN_POINT('Ctrl Pts',(3.646,-1.28099334691039,-1.16260978006393));
#22452=CARTESIAN_POINT('Ctrl Pts',(3.646,-1.27439565977673,-1.17192623953817));
#22453=CARTESIAN_POINT('Ctrl Pts',(3.646,-1.26770344996135,-1.18117916964538));
#22454=CARTESIAN_POINT('Ctrl Pts',(3.646,-1.26092631253354,-1.1903547340509));
#22455=CARTESIAN_POINT('Ctrl Pts',(3.646,-1.22063806006406,-1.24490098742961));
#22456=CARTESIAN_POINT('Ctrl Pts',(3.646,-1.17727779039597,-1.2968210133787));
#22457=CARTESIAN_POINT('Ctrl Pts',(3.646,-1.13102406755431,-1.34578478738438));
#22458=CARTESIAN_POINT('Ctrl Pts',(3.646,-1.10889356311025,-1.36921193987413));
#22459=CARTESIAN_POINT('Ctrl Pts',(3.646,-1.08609991322821,-1.39196224634769));
#22460=CARTESIAN_POINT('Ctrl Pts',(3.646,-1.06265860358067,-1.41399845269635));
#22461=CARTESIAN_POINT('Ctrl Pts',(3.646,-1.01519019024582,-1.45862154615905));
#22462=CARTESIAN_POINT('Ctrl Pts',(3.646,-0.965068683520578,-1.50031866495972));
#22463=CARTESIAN_POINT('Ctrl Pts',(3.646,-0.912608878859399,-1.53907430433262));
#22464=CARTESIAN_POINT('Ctrl Pts',(3.646,-0.885622701907269,-1.55901083571632));
#22465=CARTESIAN_POINT('Ctrl Pts',(3.646,-0.858017059499759,-1.57816846922923));
#22466=CARTESIAN_POINT('Ctrl Pts',(3.646,-0.829830930562831,-1.59654158274954));
#22467=CARTESIAN_POINT('Ctrl Pts',(3.646,-0.814618170658192,-1.6064580123987));
#22468=CARTESIAN_POINT('Ctrl Pts',(3.646,-0.799236272325966,-1.61614586579418));
#22469=CARTESIAN_POINT('Ctrl Pts',(3.646,-0.783691102223765,-1.62560394324042));
#22470=CARTESIAN_POINT('Ctrl Pts',(3.646,-0.774136405388099,-1.63141726416602));
#22471=CARTESIAN_POINT('Ctrl Pts',(3.646,-0.764521109964347,-1.63714302305682));
#22472=CARTESIAN_POINT('Ctrl Pts',(3.646,-0.754857428305642,-1.64277491414178));
#22473=CARTESIAN_POINT('Ctrl Pts',(3.646,-0.696336086560278,-1.67688053087207));
#22474=CARTESIAN_POINT('Ctrl Pts',(3.646,-0.635940296883035,-1.70761001018091));
#22475=CARTESIAN_POINT('Ctrl Pts',(3.646,-0.574032023975561,-1.73496968591445));
#22476=CARTESIAN_POINT('Ctrl Pts',(3.646,-0.510809778563976,-1.76291005724725));
#22477=CARTESIAN_POINT('Ctrl Pts',(3.646,-0.44600942822765,-1.78733655318714));
#22478=CARTESIAN_POINT('Ctrl Pts',(3.646,-0.379975375970469,-1.80821892080948));
#22479=CARTESIAN_POINT('Ctrl Pts',(3.646,-0.313405396837469,-1.82927076799057));
#22480=CARTESIAN_POINT('Ctrl Pts',(3.646,-0.245580690800976,-1.84672118374022));
#22481=CARTESIAN_POINT('Ctrl Pts',(3.646,-0.176825498658314,-1.8604948666779));
#22482=CARTESIAN_POINT('Ctrl Pts',(3.646,-0.159462280356867,-1.86397322891076));
#22483=CARTESIAN_POINT('Ctrl Pts',(3.646,-0.14203961847147,-1.86721686959177));
#22484=CARTESIAN_POINT('Ctrl Pts',(3.646,-0.124562559998911,-1.87022407918187));
#22485=CARTESIAN_POINT('Ctrl Pts',(3.646,-0.111792875781347,-1.87242130916207));
#22486=CARTESIAN_POINT('Ctrl Pts',(3.646,-0.0989925581628777,-1.87449245974032));
#22487=CARTESIAN_POINT('Ctrl Pts',(3.646,-0.0861825093113372,-1.87643420987567));
#22488=CARTESIAN_POINT('Ctrl Pts',(3.646,-0.0148835153063319,-1.88724172769734));
#22489=CARTESIAN_POINT('Ctrl Pts',(3.646,0.0568426981623723,-1.89406743257586));
#22490=CARTESIAN_POINT('Ctrl Pts',(3.646,0.128627456019564,-1.89688915407946));
#22491=CARTESIAN_POINT('Ctrl Pts',(3.646,0.200626979511061,-1.89971931760928));
#22492=CARTESIAN_POINT('Ctrl Pts',(3.646,0.272686413280953,-1.89852190431662));
#22493=CARTESIAN_POINT('Ctrl Pts',(3.646,0.344457463266169,-1.89322793788438));
#22494=CARTESIAN_POINT('Ctrl Pts',(3.646,0.414769043130747,-1.88804162468877));
#22495=CARTESIAN_POINT('Ctrl Pts',(3.646,0.484804859069096,-1.87892387244832));
#22496=CARTESIAN_POINT('Ctrl Pts',(3.646,0.554245063947006,-1.86576101897151));
#22497=CARTESIAN_POINT('Ctrl Pts',(3.646,0.579342242418372,-1.86100368158346));
#22498=CARTESIAN_POINT('Ctrl Pts',(3.646,0.60436161907656,-1.85571746700255));
#22499=CARTESIAN_POINT('Ctrl Pts',(3.646,0.629287956476874,-1.84989531266857));
#22500=CARTESIAN_POINT('',(3.646,-1.954,-2.39295984553393E-16));
#22501=CARTESIAN_POINT('Origin',(3.646,0.,0.));
#22502=CARTESIAN_POINT('',(3.646,1.85122479320614,-0.632364557278426));
#22503=CARTESIAN_POINT('Origin',(3.646,0.,0.));
#22504=CARTESIAN_POINT('Ctrl Pts',(3.646,1.85122479320614,-0.632364557278413));
#22505=CARTESIAN_POINT('Ctrl Pts',(3.646,1.86777728496137,-0.56405200123613));
#22506=CARTESIAN_POINT('Ctrl Pts',(3.646,1.88043336182538,-0.494993211783664));
#22507=CARTESIAN_POINT('Ctrl Pts',(3.646,1.88896124154753,-0.425422790109387));
#22508=CARTESIAN_POINT('Ctrl Pts',(3.646,1.88988050194317,-0.41792346607611));
#22509=CARTESIAN_POINT('Ctrl Pts',(3.646,1.89075174381644,-0.410418197460951));
#22510=CARTESIAN_POINT('Ctrl Pts',(3.646,1.89157464001029,-0.402907279500277));
#22511=CARTESIAN_POINT('Ctrl Pts',(3.646,1.89970424140916,-0.328705005123505));
#22512=CARTESIAN_POINT('Ctrl Pts',(3.646,1.90312005139857,-0.253949891494488));
#22513=CARTESIAN_POINT('Ctrl Pts',(3.646,1.90195657636727,-0.179041257804402));
#22514=CARTESIAN_POINT('Ctrl Pts',(3.646,1.90168714256733,-0.161694157711369));
#22515=CARTESIAN_POINT('Ctrl Pts',(3.646,1.9011718953687,-0.144338912994997));
#22516=CARTESIAN_POINT('Ctrl Pts',(3.646,1.90041209170278,-0.126980670648089));
#22517=CARTESIAN_POINT('Ctrl Pts',(3.646,1.89981112648655,-0.113251202979906));
#22518=CARTESIAN_POINT('Ctrl Pts',(3.646,1.89905757038205,-0.099529250292602));
#22519=CARTESIAN_POINT('Ctrl Pts',(3.646,1.89815266633269,-0.0858180755197819));
#22520=CARTESIAN_POINT('Ctrl Pts',(3.646,1.89346054585753,-0.0147227102867202));
#22521=CARTESIAN_POINT('Ctrl Pts',(3.646,1.88470293100181,0.0560916653141868));
#22522=CARTESIAN_POINT('Ctrl Pts',(3.646,1.87201708655583,0.126279358269305));
#22523=CARTESIAN_POINT('Ctrl Pts',(3.646,1.86260788358229,0.178338190621555));
#22524=CARTESIAN_POINT('Ctrl Pts',(3.646,1.851036486259,0.230052140379478));
#22525=CARTESIAN_POINT('Ctrl Pts',(3.646,1.83734247846642,0.281271602238531));
#22526=CARTESIAN_POINT('Ctrl Pts',(3.646,1.83198896790198,0.301295245741617));
#22527=CARTESIAN_POINT('Ctrl Pts',(3.646,1.82631091397735,0.321243214387335));
#22528=CARTESIAN_POINT('Ctrl Pts',(3.646,1.82031016933083,0.341106135959376));
#22529=CARTESIAN_POINT('Ctrl Pts',(3.646,1.81552257077984,0.356953451607448));
#22530=CARTESIAN_POINT('Ctrl Pts',(3.646,1.81052809968397,0.372750635976576));
#22531=CARTESIAN_POINT('Ctrl Pts',(3.646,1.80533673969134,0.388466303818269));
#22532=CARTESIAN_POINT('Ctrl Pts',(3.646,1.78349989834249,0.454572400455262));
#22533=CARTESIAN_POINT('Ctrl Pts',(3.646,1.75815877282522,0.519325115466895));
#22534=CARTESIAN_POINT('Ctrl Pts',(3.646,1.72944007783936,0.582403703796427));
#22535=CARTESIAN_POINT('Ctrl Pts',(3.646,1.7013580179239,0.644083968088538));
#22536=CARTESIAN_POINT('Ctrl Pts',(3.646,1.67004582822095,0.704164273758678));
#22537=CARTESIAN_POINT('Ctrl Pts',(3.646,1.63558364196677,0.762314720566202));
#22538=CARTESIAN_POINT('Ctrl Pts',(3.646,1.6107204306916,0.804268148420632));
#22539=CARTESIAN_POINT('Ctrl Pts',(3.646,1.58421680890061,0.845216482048597));
#22540=CARTESIAN_POINT('Ctrl Pts',(3.646,1.55609275564537,0.885022483158703));
#22541=CARTESIAN_POINT('Ctrl Pts',(3.646,1.54206067170508,0.904883103668667));
#22542=CARTESIAN_POINT('Ctrl Pts',(3.646,1.52762508230321,0.924459162026505));
#22543=CARTESIAN_POINT('Ctrl Pts',(3.646,1.51278780298836,0.943732354103002));
#22544=CARTESIAN_POINT('Ctrl Pts',(3.646,1.5040149219818,0.955128070063854));
#22545=CARTESIAN_POINT('Ctrl Pts',(3.646,1.49510160076979,0.966417886209972));
#22546=CARTESIAN_POINT('Ctrl Pts',(3.646,1.48604814989002,0.977597866731241));
#22547=CARTESIAN_POINT('Ctrl Pts',(3.646,1.47811974575181,0.987388542685312));
#22548=CARTESIAN_POINT('Ctrl Pts',(3.646,1.4700886402459,0.997089004542171));
#22549=CARTESIAN_POINT('Ctrl Pts',(3.646,1.46196065824995,1.00669091177099));
#22550=CARTESIAN_POINT('Ctrl Pts',(3.646,1.4198448625495,1.05644397020358));
#22551=CARTESIAN_POINT('Ctrl Pts',(3.646,1.37508773873266,1.10360721210258));
#22552=CARTESIAN_POINT('Ctrl Pts',(3.646,1.32776700421932,1.14788094866693));
#22553=CARTESIAN_POINT('Ctrl Pts',(3.646,1.30623682000847,1.16802479710327));
#22554=CARTESIAN_POINT('Ctrl Pts',(3.646,1.28417551167546,1.18756994121615));
#22555=CARTESIAN_POINT('Ctrl Pts',(3.646,1.26158843649361,1.20648512205778));
#22556=CARTESIAN_POINT('Ctrl Pts',(3.646,1.21030221098365,1.24943394223017));
#22557=CARTESIAN_POINT('Ctrl Pts',(3.646,1.15630601551353,1.28913837264243));
#22558=CARTESIAN_POINT('Ctrl Pts',(3.646,1.09994475084755,1.32549904345976));
#22559=CARTESIAN_POINT('Ctrl Pts',(3.646,1.07528669755618,1.34140683694234));
#22560=CARTESIAN_POINT('Ctrl Pts',(3.646,1.05017579133236,1.35667393594728));
#22561=CARTESIAN_POINT('Ctrl Pts',(3.646,1.0246405521453,1.37128880994725));
#22562=CARTESIAN_POINT('Ctrl Pts',(3.646,1.00962813908413,1.37988103513524));
#22563=CARTESIAN_POINT('Ctrl Pts',(3.646,0.99446905996368,1.38824778952788));
#22564=CARTESIAN_POINT('Ctrl Pts',(3.646,0.97916913378863,1.39638640825901));
#22565=CARTESIAN_POINT('Ctrl Pts',(3.646,0.968921661455415,1.40183743261845));
#22566=CARTESIAN_POINT('Ctrl Pts',(3.646,0.958610248820093,1.40718638752318));
#22567=CARTESIAN_POINT('Ctrl Pts',(3.646,0.948251329433642,1.41242531107771));
#22568=CARTESIAN_POINT('Ctrl Pts',(3.646,0.890485005097459,1.44164007237986));
#22569=CARTESIAN_POINT('Ctrl Pts',(3.646,0.831136756612497,1.46749477000214));
#22570=CARTESIAN_POINT('Ctrl Pts',(3.646,0.770533170445064,1.48993478777504));
#22571=CARTESIAN_POINT('Ctrl Pts',(3.646,0.71007092264702,1.51232247142513));
#22572=CARTESIAN_POINT('Ctrl Pts',(3.646,0.648358055128917,1.53131144137255));
#22573=CARTESIAN_POINT('Ctrl Pts',(3.646,0.585713135036152,1.54679634298933));
#22574=CARTESIAN_POINT('Ctrl Pts',(3.646,0.524282126391685,1.5619811835745));
#22575=CARTESIAN_POINT('Ctrl Pts',(3.646,0.461953855213984,1.57379634993966));
#22576=CARTESIAN_POINT('Ctrl Pts',(3.646,0.399038762127085,1.58209375444539));
#22577=CARTESIAN_POINT('Ctrl Pts',(3.646,0.385552018248948,1.58387242096135));
#22578=CARTESIAN_POINT('Ctrl Pts',(3.646,0.372038376342684,1.5854892608117));
#22579=CARTESIAN_POINT('Ctrl Pts',(3.646,0.358501021440916,1.58694252210702));
#22580=CARTESIAN_POINT('Ctrl Pts',(3.646,0.347711851978039,1.58810076036721));
#22581=CARTESIAN_POINT('Ctrl Pts',(3.646,0.336912962054473,1.58915446959528));
#22582=CARTESIAN_POINT('Ctrl Pts',(3.646,0.326113495044186,1.59010251750235));
#22583=CARTESIAN_POINT('Ctrl Pts',(3.646,0.264279472447157,1.59553071276911));
#22584=CARTESIAN_POINT('Ctrl Pts',(3.646,0.202349440359449,1.59750742949326));
#22585=CARTESIAN_POINT('Ctrl Pts',(3.646,0.140612115364729,1.59594625728721));
#22586=CARTESIAN_POINT('Ctrl Pts',(3.646,0.0799615604267115,1.5944125665959));
#22587=CARTESIAN_POINT('Ctrl Pts',(3.646,0.0194961016000075,1.58946431823579));
#22588=CARTESIAN_POINT('Ctrl Pts',(3.646,-0.0404959561586677,1.5809719777752));
#22589=CARTESIAN_POINT('Ctrl Pts',(3.646,-0.0985852921086698,1.57274898232468));
#22590=CARTESIAN_POINT('Ctrl Pts',(3.646,-0.156231425499309,1.561202914565));
#22591=CARTESIAN_POINT('Ctrl Pts',(3.646,-0.213147860982218,1.54617388631109));
#22592=CARTESIAN_POINT('Ctrl Pts',(3.646,-0.227131809032557,1.54248136501093));
#22593=CARTESIAN_POINT('Ctrl Pts',(3.646,-0.24107156350228,1.53857839846659));
#22594=CARTESIAN_POINT('Ctrl Pts',(3.646,-0.254962570226321,1.53446223081039));
#22595=CARTESIAN_POINT('Ctrl Pts',(0.178525917727935,-0.685825729128712,
1.39614588036676));
#22596=CARTESIAN_POINT('Ctrl Pts',(0.214645439418269,-1.13846748842057,
1.17379564536202));
#22597=CARTESIAN_POINT('Ctrl Pts',(0.286884482798937,-1.80431739237854,
0.259468333747379));
#22598=CARTESIAN_POINT('Ctrl Pts',(0.395243047869939,-1.22944579344352,
-1.34783917131191));
#22599=CARTESIAN_POINT('Ctrl Pts',(0.503601612940941,0.420984007196011,
-1.77351976747628));
#22600=CARTESIAN_POINT('Ctrl Pts',(0.611960178011943,1.70289301291901,-0.651599460365548));
#22601=CARTESIAN_POINT('Ctrl Pts',(0.720318743082945,1.49728705490344,1.04067255962924));
#22602=CARTESIAN_POINT('Ctrl Pts',(0.828677308153947,-0.0167383245662881,
1.8231374532372));
#22603=CARTESIAN_POINT('Ctrl Pts',(0.937035873224949,-1.51604025138297,
1.0129450519225));
#22604=CARTESIAN_POINT('Ctrl Pts',(1.04539443829595,-1.69077758585837,-0.682438578679264));
#22605=CARTESIAN_POINT('Ctrl Pts',(1.15375300336695,-0.388197806685981,
-1.78147566906063));
#22606=CARTESIAN_POINT('Ctrl Pts',(1.26211156843795,1.2535495552727,-1.3240166887812));
#22607=CARTESIAN_POINT('Ctrl Pts',(1.37047013350896,1.8000352141881,0.290301877450055));
#22608=CARTESIAN_POINT('Ctrl Pts',(1.47882869857996,0.773764763351813,1.65096279999703));
#22609=CARTESIAN_POINT('Ctrl Pts',(1.58718726365096,-0.928568406390638,
1.56912687330982));
#22610=CARTESIAN_POINT('Ctrl Pts',(1.69554582872196,-1.81958063721889,0.11628815110578));
#22611=CARTESIAN_POINT('Ctrl Pts',(1.80390439379297,-1.1207626488587,-1.43815386147426));
#22612=CARTESIAN_POINT('Ctrl Pts',(1.91226295886397,0.557303862904986,-1.73603266764626));
#22613=CARTESIAN_POINT('Ctrl Pts',(2.02062152393497,1.74843472771405,-0.517079730093531));
#22614=CARTESIAN_POINT('Ctrl Pts',(2.12898008900597,1.41189906885343,1.15366271015419));
#22615=CARTESIAN_POINT('Ctrl Pts',(2.23733865407697,-0.158262365011203,
1.81641169719614));
#22616=CARTESIAN_POINT('Ctrl Pts',(2.34569721914797,-1.59014198076045,0.892097840487327));
#22617=CARTESIAN_POINT('Ctrl Pts',(2.45405578421898,-1.63266518861614,-0.811668857508549));
#22618=CARTESIAN_POINT('Ctrl Pts',(2.56241434928998,-0.248663526484289,
-1.80625943050602));
#22619=CARTESIAN_POINT('Ctrl Pts',(2.67077291436098,1.35258575494928,-1.22264666689896));
#22620=CARTESIAN_POINT('Ctrl Pts',(2.77913147943198,1.77206945169698,0.429209875088153));
#22621=CARTESIAN_POINT('Ctrl Pts',(2.88749004450298,0.643168985847878,1.70609770460869));
#22622=CARTESIAN_POINT('Ctrl Pts',(2.99584860957399,-1.04756297297815,1.4922205475568));
#22623=CARTESIAN_POINT('Ctrl Pts',(3.10420717464499,-1.82324663843674,-0.0252902466545985));
#22624=CARTESIAN_POINT('Ctrl Pts',(3.21256573971599,-1.00543213394195,-1.52103014244754));
#22625=CARTESIAN_POINT('Ctrl Pts',(3.320924304787,0.68997158388018,-1.68716896408801));
#22626=CARTESIAN_POINT('Ctrl Pts',(3.429282869858,1.78424156303041,-0.380380645529688));
#22627=CARTESIAN_POINT('Ctrl Pts',(3.53764143492899,1.31614849123568,1.26120506567147));
#22628=CARTESIAN_POINT('Ctrl Pts',(3.60988047830967,0.242522465892156,1.61712315325676));
#22629=CARTESIAN_POINT('Ctrl Pts',(3.646,-0.254962570226321,1.53446223081039));
#22630=CARTESIAN_POINT('Ctrl Pts',(0.25521727848529,-0.744392439309316,
1.51537102412035));
#22631=CARTESIAN_POINT('Ctrl Pts',(0.291336800175624,-1.23568795218047,
1.27403298912647));
#22632=CARTESIAN_POINT('Ctrl Pts',(0.363575843556292,-1.95839871261059,
0.281625867444654));
#22633=CARTESIAN_POINT('Ctrl Pts',(0.471934408627294,-1.33443543207789,
-1.46293911983174));
#22634=CARTESIAN_POINT('Ctrl Pts',(0.580292973698296,0.456934318321611,
-1.92497109659646));
#22635=CARTESIAN_POINT('Ctrl Pts',(0.688651538769298,1.84831310627553,-0.707243387282011));
#22636=CARTESIAN_POINT('Ctrl Pts',(0.7970101038403,1.62514924099131,1.12954173674534));
#22637=CARTESIAN_POINT('Ctrl Pts',(0.905368668911302,-0.0181677089742313,
1.97882592963601));
#22638=CARTESIAN_POINT('Ctrl Pts',(1.0137272339823,-1.64550388369329,1.09944641336922));
#22639=CARTESIAN_POINT('Ctrl Pts',(1.12208579905331,-1.8351630713324,-0.740716040075106));
#22640=CARTESIAN_POINT('Ctrl Pts',(1.23044436412431,-0.421348310482051,
-1.93360639961257));
#22641=CARTESIAN_POINT('Ctrl Pts',(1.33880292919531,1.36059755651049,-1.43708229479842));
#22642=CARTESIAN_POINT('Ctrl Pts',(1.44716149426631,1.95375085392965,0.315092469577743));
#22643=CARTESIAN_POINT('Ctrl Pts',(1.55552005933731,0.83984110712031,1.79194826572055));
#22644=CARTESIAN_POINT('Ctrl Pts',(1.66387862440832,-1.00786434766282,1.70312388584898));
#22645=CARTESIAN_POINT('Ctrl Pts',(1.77223718947932,-1.9749653760878,0.126218683242426));
#22646=CARTESIAN_POINT('Ctrl Pts',(1.88059575455032,-1.21647119178599,-1.56096631487563));
#22647=CARTESIAN_POINT('Ctrl Pts',(1.98895431962132,0.604895331750507,-1.88428275187577));
#22648=CARTESIAN_POINT('Ctrl Pts',(2.09731288469232,1.89774389711168,-0.561236222634466));
#22649=CARTESIAN_POINT('Ctrl Pts',(2.20567144976333,1.53246947042594,1.25218078365605));
#22650=CARTESIAN_POINT('Ctrl Pts',(2.31403001483433,-0.171777323214773,
1.97152582155758));
#22651=CARTESIAN_POINT('Ctrl Pts',(2.42238857990533,-1.72593359746098,0.96827934470552));
#22652=CARTESIAN_POINT('Ctrl Pts',(2.53074714497633,-1.77208811321992,-0.880982055776449));
#22653=CARTESIAN_POINT('Ctrl Pts',(2.63910571004733,-0.269898373865409,
-1.96050659284538));
#22654=CARTESIAN_POINT('Ctrl Pts',(2.74746427511834,1.46809104228396,-1.32705568795526));
#22655=CARTESIAN_POINT('Ctrl Pts',(2.85582284018934,1.92339692978575,0.465862641663236));
#22656=CARTESIAN_POINT('Ctrl Pts',(2.96418140526034,0.698092984746491,1.8517914655187));
#22657=CARTESIAN_POINT('Ctrl Pts',(3.07253997033134,-1.13702056319175,1.61965007465449));
#22658=CARTESIAN_POINT('Ctrl Pts',(3.18089853540234,-1.97894443880469,-0.0274499302058373));
#22659=CARTESIAN_POINT('Ctrl Pts',(3.28925710047335,-1.09129192294352,-1.65091989103114));
#22660=CARTESIAN_POINT('Ctrl Pts',(3.39761566554435,0.748892333087561,-1.83124628803295));
#22661=CARTESIAN_POINT('Ctrl Pts',(3.50597423061535,1.93660848960656,-0.412863595758679));
#22662=CARTESIAN_POINT('Ctrl Pts',(3.61433279568635,1.42854218538706,1.36890681616329));
#22663=CARTESIAN_POINT('Ctrl Pts',(3.68657183906702,0.263232891834088,1.75521885165445));
#22664=CARTESIAN_POINT('Ctrl Pts',(3.72269136075735,-0.276735330161002,
1.66549902476259));
#22665=CARTESIAN_POINT('Ctrl Pts',(0.331908639242645,-0.80295914948992,
1.63459616787395));
#22666=CARTESIAN_POINT('Ctrl Pts',(0.368028160932979,-1.33290841594038,
1.37427033289091));
#22667=CARTESIAN_POINT('Ctrl Pts',(0.440267204313648,-2.11248003284263,
0.303783401141929));
#22668=CARTESIAN_POINT('Ctrl Pts',(0.548625769384649,-1.43942507071225,
-1.57803906835158));
#22669=CARTESIAN_POINT('Ctrl Pts',(0.656984334455651,0.492884629447209,
-2.07642242571663));
#22670=CARTESIAN_POINT('Ctrl Pts',(0.765342899526654,1.99373319963206,-0.762887314198474));
#22671=CARTESIAN_POINT('Ctrl Pts',(0.873701464597655,1.75301142707918,1.21841091386143));
#22672=CARTESIAN_POINT('Ctrl Pts',(0.982060029668658,-0.0195970933821744,
2.13451440603482));
#22673=CARTESIAN_POINT('Ctrl Pts',(1.09041859473966,-1.77496751600361,1.18594777481594));
#22674=CARTESIAN_POINT('Ctrl Pts',(1.19877715981066,-1.97954855680643,-0.798993501470944));
#22675=CARTESIAN_POINT('Ctrl Pts',(1.30713572488166,-0.454498814278123,
-2.08573713016452));
#22676=CARTESIAN_POINT('Ctrl Pts',(1.41549428995266,1.46764555774828,-1.55014790081563));
#22677=CARTESIAN_POINT('Ctrl Pts',(1.52385285502367,2.10746649367121,0.339883061705427));
#22678=CARTESIAN_POINT('Ctrl Pts',(1.63221142009467,0.905917450888808,1.93293373144407));
#22679=CARTESIAN_POINT('Ctrl Pts',(1.74056998516567,-1.08716028893501,1.83712089838813));
#22680=CARTESIAN_POINT('Ctrl Pts',(1.84892855023667,-2.1303501149567,0.136149215379072));
#22681=CARTESIAN_POINT('Ctrl Pts',(1.95728711530768,-1.31217973471328,-1.683778768277));
#22682=CARTESIAN_POINT('Ctrl Pts',(2.06564568037868,0.652486800596032,-2.03253283610529));
#22683=CARTESIAN_POINT('Ctrl Pts',(2.17400424544968,2.04705306650931,-0.605392715175402));
#22684=CARTESIAN_POINT('Ctrl Pts',(2.28236281052068,1.65303987199845,1.35069885715791));
#22685=CARTESIAN_POINT('Ctrl Pts',(2.39072137559168,-0.185292281418345,
2.12663994591902));
#22686=CARTESIAN_POINT('Ctrl Pts',(2.49907994066268,-1.86172521416151,1.04446084892372));
#22687=CARTESIAN_POINT('Ctrl Pts',(2.60743850573369,-1.9115110378237,-0.95029525404435));
#22688=CARTESIAN_POINT('Ctrl Pts',(2.71579707080469,-0.291133221246527,
-2.11475375518475));
#22689=CARTESIAN_POINT('Ctrl Pts',(2.8241556358757,1.58359632961863,-1.43146470901156));
#22690=CARTESIAN_POINT('Ctrl Pts',(2.93251420094669,2.07472440787453,0.502515408238319));
#22691=CARTESIAN_POINT('Ctrl Pts',(3.04087276601769,0.753016983645105,1.99748522642871));
#22692=CARTESIAN_POINT('Ctrl Pts',(3.1492313310887,-1.22647815340536,1.74707960175219));
#22693=CARTESIAN_POINT('Ctrl Pts',(3.2575898961597,-2.13464223917264,-0.029609613757076));
#22694=CARTESIAN_POINT('Ctrl Pts',(3.3659484612307,-1.1771517119451,-1.78080963961473));
#22695=CARTESIAN_POINT('Ctrl Pts',(3.4743070263017,0.807813082294942,-1.9753236119779));
#22696=CARTESIAN_POINT('Ctrl Pts',(3.58266559137271,2.08897541618271,-0.44534654598767));
#22697=CARTESIAN_POINT('Ctrl Pts',(3.69102415644371,1.54093587953844,1.47660856665511));
#22698=CARTESIAN_POINT('Ctrl Pts',(3.76326319982438,0.283943317776021,1.89331455005214));
#22699=CARTESIAN_POINT('Ctrl Pts',(3.79938272151471,-0.298508090095682,
1.79653581871479));
#22700=CARTESIAN_POINT('Ctrl Pts',(0.408600000000001,-0.861525859670525,
1.75382131162755));
#22701=CARTESIAN_POINT('Ctrl Pts',(0.444719521690335,-1.43012887970028,
1.47450767665535));
#22702=CARTESIAN_POINT('Ctrl Pts',(0.516958565071002,-2.26656135307468,
0.325940934839204));
#22703=CARTESIAN_POINT('Ctrl Pts',(0.625317130142005,-1.54441470934661,
-1.69313901687141));
#22704=CARTESIAN_POINT('Ctrl Pts',(0.733675695213006,0.528834940572807,
-2.22787375483681));
#22705=CARTESIAN_POINT('Ctrl Pts',(0.84203426028401,2.13915329298858,-0.818531241114937));
#22706=CARTESIAN_POINT('Ctrl Pts',(0.950392825355009,1.88087361316704,1.30728009097753));
#22707=CARTESIAN_POINT('Ctrl Pts',(1.05875139042601,-0.0210264777901153,
2.29020288243362));
#22708=CARTESIAN_POINT('Ctrl Pts',(1.16710995549701,-1.90443114831393,1.27244913626267));
#22709=CARTESIAN_POINT('Ctrl Pts',(1.27546852056802,-2.12393404228046,-0.857270962866784));
#22710=CARTESIAN_POINT('Ctrl Pts',(1.38382708563902,-0.487649318074194,
-2.23786786071647));
#22711=CARTESIAN_POINT('Ctrl Pts',(1.49218565071002,1.57469355898608,-1.66321350683284));
#22712=CARTESIAN_POINT('Ctrl Pts',(1.60054421578102,2.26118213341276,0.364673653833113));
#22713=CARTESIAN_POINT('Ctrl Pts',(1.70890278085203,0.971993794657307,2.07391919716759));
#22714=CARTESIAN_POINT('Ctrl Pts',(1.81726134592303,-1.1664562302072,1.97111791092728));
#22715=CARTESIAN_POINT('Ctrl Pts',(1.92561991099403,-2.2857348538256,0.146079747515718));
#22716=CARTESIAN_POINT('Ctrl Pts',(2.03397847606503,-1.40788827764057,-1.80659122167837));
#22717=CARTESIAN_POINT('Ctrl Pts',(2.14233704113603,0.700078269441555,-2.1807829203348));
#22718=CARTESIAN_POINT('Ctrl Pts',(2.25069560620703,2.19636223590694,-0.649549207716336));
#22719=CARTESIAN_POINT('Ctrl Pts',(2.35905417127804,1.77361027357095,1.44921693065978));
#22720=CARTESIAN_POINT('Ctrl Pts',(2.46741273634904,-0.198807239621914,
2.28175407028046));
#22721=CARTESIAN_POINT('Ctrl Pts',(2.57577130142004,-1.99751683086205,1.12064235314191));
#22722=CARTESIAN_POINT('Ctrl Pts',(2.68412986649105,-2.05093396242748,-1.01960845231225));
#22723=CARTESIAN_POINT('Ctrl Pts',(2.79248843156204,-0.312368068627645,
-2.26900091752411));
#22724=CARTESIAN_POINT('Ctrl Pts',(2.90084699663305,1.69910161695331,-1.53587373006786));
#22725=CARTESIAN_POINT('Ctrl Pts',(3.00920556170405,2.2260518859633,0.539168174813403));
#22726=CARTESIAN_POINT('Ctrl Pts',(3.11756412677505,0.807940982543718,2.14317898733871));
#22727=CARTESIAN_POINT('Ctrl Pts',(3.22592269184605,-1.31593574361896,1.87450912884988));
#22728=CARTESIAN_POINT('Ctrl Pts',(3.33428125691705,-2.29034003954059,-0.0317692973083151));
#22729=CARTESIAN_POINT('Ctrl Pts',(3.44263982198806,-1.26301150094668,-1.91069938819832));
#22730=CARTESIAN_POINT('Ctrl Pts',(3.55099838705906,0.866733831502324,-2.11940093592284));
#22731=CARTESIAN_POINT('Ctrl Pts',(3.65935695213006,2.24134234275887,-0.477829496216659));
#22732=CARTESIAN_POINT('Ctrl Pts',(3.76771551720106,1.65332957368982,1.58431031714693));
#22733=CARTESIAN_POINT('Ctrl Pts',(3.83995456058173,0.304653743717953,2.03141024844982));
#22734=CARTESIAN_POINT('Ctrl Pts',(3.87607408227206,-0.320280850030362,
1.92757261266699));
#22735=CARTESIAN_POINT('Ctrl Pts',(3.33273030787577,-1.95689202958038,-0.000120183693368507));
#22736=CARTESIAN_POINT('Ctrl Pts',(3.33324729088953,-1.95690205649134,-0.00915092760564931));
#22737=CARTESIAN_POINT('Ctrl Pts',(3.33376427390329,-1.95684415228561,-0.0181815514118841));
#22738=CARTESIAN_POINT('Ctrl Pts',(3.33428125691705,-1.95671790045467,-0.0272112414302843));
#22739=CARTESIAN_POINT('Ctrl Pts',(3.37040077860739,-1.94789719334262,-0.658079327604984));
#22740=CARTESIAN_POINT('Ctrl Pts',(3.40652030029772,-1.60545434714465,-1.28438935790166));
#22741=CARTESIAN_POINT('Ctrl Pts',(3.44263982198806,-1.0792753686375,-1.63232796433741));
#22742=CARTESIAN_POINT('Ctrl Pts',(3.47875934367839,-0.553096390130347,
-1.98026657077316));
#22743=CARTESIAN_POINT('Ctrl Pts',(3.51487886536873,0.156818720685984,-2.049833753348));
#22744=CARTESIAN_POINT('Ctrl Pts',(3.55099838705906,0.740877694636909,-1.81102210468439));
#22745=CARTESIAN_POINT('Ctrl Pts',(3.58266559137271,1.2529419190165,-1.60164786834911));
#22746=CARTESIAN_POINT('Ctrl Pts',(3.61433279568635,1.668265301163,-1.1552345125566));
#22747=CARTESIAN_POINT('Ctrl Pts',(3.646,1.85122479320614,-0.632364557278426));
#22748=CARTESIAN_POINT('',(0.408600000000001,-0.905313301390919,-1.26710934922959));
#22749=CARTESIAN_POINT('Ctrl Pts',(0.408600000000001,-0.905313301390914,
-1.26710934922959));
#22750=CARTESIAN_POINT('Ctrl Pts',(0.408600000000001,-0.960992218100913,
-1.23747014056059));
#22751=CARTESIAN_POINT('Ctrl Pts',(0.4086,-1.0146111721236,-1.20440946055571));
#22752=CARTESIAN_POINT('Ctrl Pts',(0.4086,-1.06580548946931,-1.16801868547721));
#22753=CARTESIAN_POINT('Ctrl Pts',(0.408600000000001,-1.11460808220303,
-1.13332803488357));
#22754=CARTESIAN_POINT('Ctrl Pts',(0.408600000000001,-1.16120868065023,
-1.09561111056787));
#22755=CARTESIAN_POINT('Ctrl Pts',(0.408600000000001,-1.20553237586123,
-1.05517990554672));
#22756=CARTESIAN_POINT('Ctrl Pts',(0.408600000000001,-1.21581352958369,
-1.04580163886502));
#22757=CARTESIAN_POINT('Ctrl Pts',(0.408600000000001,-1.22597208544125,
-1.03627713244074));
#22758=CARTESIAN_POINT('Ctrl Pts',(0.408600000000001,-1.23600692964817,
-1.02660993024093));
#22759=CARTESIAN_POINT('Ctrl Pts',(0.408600000000001,-1.24536959860237,
-1.01759027711592));
#22760=CARTESIAN_POINT('Ctrl Pts',(0.408600000000001,-1.25462100326372,
-1.0084497486066));
#22761=CARTESIAN_POINT('Ctrl Pts',(0.408600000000001,-1.2637547881083,-0.999197404829853));
#22762=CARTESIAN_POINT('Ctrl Pts',(0.408600000000001,-1.30741516684387,
-0.954970302882759));
#22763=CARTESIAN_POINT('Ctrl Pts',(0.408600000000001,-1.34842999904488,
-0.908153772000464));
#22764=CARTESIAN_POINT('Ctrl Pts',(0.408600000000001,-1.38672592196133,
-0.859098143986562));
#22765=CARTESIAN_POINT('Ctrl Pts',(0.408600000000001,-1.41723561179862,
-0.820016385890729));
#22766=CARTESIAN_POINT('Ctrl Pts',(0.408600000000001,-1.44601935179638,
-0.779512241439089));
#22767=CARTESIAN_POINT('Ctrl Pts',(0.408600000000001,-1.47302824589713,
-0.737742377449649));
#22768=CARTESIAN_POINT('Ctrl Pts',(0.408600000000001,-1.48400331805306,
-0.720769180786444));
#22769=CARTESIAN_POINT('Ctrl Pts',(0.408600000000001,-1.4946851893039,-0.703586803249634));
#22770=CARTESIAN_POINT('Ctrl Pts',(0.408600000000001,-1.50506997244662,
-0.686205058605768));
#22771=CARTESIAN_POINT('Ctrl Pts',(0.4086,-1.51138034557605,-0.675642941627891));
#22772=CARTESIAN_POINT('Ctrl Pts',(0.408600000000001,-1.51757627535282,
-0.665015095569133));
#22773=CARTESIAN_POINT('Ctrl Pts',(0.408600000000001,-1.52365605181011,
-0.654326316602663));
#22774=CARTESIAN_POINT('Ctrl Pts',(0.408600000000001,-1.55558277317524,
-0.598196346990612));
#22775=CARTESIAN_POINT('Ctrl Pts',(0.408600000000001,-1.5843201739237,-0.540370467208204));
#22776=CARTESIAN_POINT('Ctrl Pts',(0.408600000000001,-1.60979082996186,
-0.481204228927061));
#22777=CARTESIAN_POINT('Ctrl Pts',(0.408600000000001,-1.63580594349255,
-0.420773260688075));
#22778=CARTESIAN_POINT('Ctrl Pts',(0.408600000000001,-1.65841388453419,
-0.358943232312242));
#22779=CARTESIAN_POINT('Ctrl Pts',(0.408600000000001,-1.67749735979264,
-0.296051832948879));
#22780=CARTESIAN_POINT('Ctrl Pts',(0.408600000000001,-1.69091866366144,
-0.251820655442808));
#22781=CARTESIAN_POINT('Ctrl Pts',(0.408600000000001,-1.70259596991367,
-0.207063606073226));
#22782=CARTESIAN_POINT('Ctrl Pts',(0.408600000000001,-1.71247552643195,
-0.161889744563548));
#22783=CARTESIAN_POINT('Ctrl Pts',(0.408600000000001,-1.71825809865879,
-0.135449173424395));
#22784=CARTESIAN_POINT('Ctrl Pts',(0.408600000000001,-1.72342457757944,
-0.108865697407971));
#22785=CARTESIAN_POINT('Ctrl Pts',(0.408600000000001,-1.72796221803694,
-0.0821604924653415));
#22786=CARTESIAN_POINT('Ctrl Pts',(0.408600000000001,-1.72987457329142,
-0.0709057799176328));
#22787=CARTESIAN_POINT('Ctrl Pts',(0.408600000000001,-1.73167514932966,
-0.0596292516012904));
#22788=CARTESIAN_POINT('Ctrl Pts',(0.408600000000001,-1.73336096201533,
-0.0483474786684694));
#22789=CARTESIAN_POINT('Ctrl Pts',(0.408600000000001,-1.74338265810016,
0.0187195807926847));
#22790=CARTESIAN_POINT('Ctrl Pts',(0.408600000000001,-1.74937481327135,
0.0860982634108857));
#22791=CARTESIAN_POINT('Ctrl Pts',(0.408600000000001,-1.751230653984,0.153428852725802));
#22792=CARTESIAN_POINT('Ctrl Pts',(0.408600000000001,-1.75211859736995,
0.18564376807186));
#22793=CARTESIAN_POINT('Ctrl Pts',(0.408600000000001,-1.7520590352964,0.217848150864259));
#22794=CARTESIAN_POINT('Ctrl Pts',(0.408600000000001,-1.75103660889884,
0.250004695309369));
#22795=CARTESIAN_POINT('Ctrl Pts',(0.408600000000001,-1.74896620456347,
0.315121410985578));
#22796=CARTESIAN_POINT('Ctrl Pts',(0.408600000000001,-1.74295098459612,
0.380041655358923));
#22797=CARTESIAN_POINT('Ctrl Pts',(0.408600000000001,-1.73320278712455,
0.444532054942262));
#22798=CARTESIAN_POINT('Ctrl Pts',(0.408600000000001,-1.72818815850798,
0.47770694744813));
#22799=CARTESIAN_POINT('Ctrl Pts',(0.408600000000001,-1.72218484157449,
0.510768222096462));
#22800=CARTESIAN_POINT('Ctrl Pts',(0.408600000000001,-1.71521645115096,
0.54368436163359));
#22801=CARTESIAN_POINT('Ctrl Pts',(0.408600000000001,-1.71145543383829,
0.561450038230503));
#22802=CARTESIAN_POINT('Ctrl Pts',(0.408600000000001,-1.70741322783236,
0.579173434823943));
#22803=CARTESIAN_POINT('Ctrl Pts',(0.408600000000001,-1.70309313761823,
0.596849557588417));
#22804=CARTESIAN_POINT('Ctrl Pts',(0.408600000000001,-1.70043783745291,
0.607714009341151));
#22805=CARTESIAN_POINT('Ctrl Pts',(0.408600000000001,-1.69767778945195,
0.618559301444646));
#22806=CARTESIAN_POINT('Ctrl Pts',(0.408600000000001,-1.6948171819072,0.62937234343737));
#22807=CARTESIAN_POINT('Ctrl Pts',(0.408600000000001,-1.67749388530445,
0.694854074394054));
#22808=CARTESIAN_POINT('Ctrl Pts',(0.408600000000001,-1.65645882135167,
0.759270632936003));
#22809=CARTESIAN_POINT('Ctrl Pts',(0.408600000000001,-1.63197264004038,
0.822370777365584));
#22810=CARTESIAN_POINT('Ctrl Pts',(0.408600000000001,-1.60696675159071,
0.886810191282533));
#22811=CARTESIAN_POINT('Ctrl Pts',(0.408600000000001,-1.57836151994529,
0.94987758575432));
#22812=CARTESIAN_POINT('Ctrl Pts',(0.408600000000001,-1.5463793183319,1.01130823187454));
#22813=CARTESIAN_POINT('Ctrl Pts',(0.408600000000001,-1.51413756653462,
1.07323741576553));
#22814=CARTESIAN_POINT('Ctrl Pts',(0.408600000000001,-1.47846348459479,
1.13350415064642));
#22815=CARTESIAN_POINT('Ctrl Pts',(0.408600000000001,-1.43953335033057,
1.19182606932565));
#22816=CARTESIAN_POINT('Ctrl Pts',(0.408600000000001,-1.42970202868341,
1.20655454515683));
#22817=CARTESIAN_POINT('Ctrl Pts',(0.408600000000001,-1.41966281092328,
1.22115889316257));
#22818=CARTESIAN_POINT('Ctrl Pts',(0.408600000000001,-1.40941806125765,
1.23563433772608));
#22819=CARTESIAN_POINT('Ctrl Pts',(0.408600000000001,-1.401932841117,1.24621067123621));
#22820=CARTESIAN_POINT('Ctrl Pts',(0.408600000000001,-1.39433687267044,
1.25671941680317));
#22821=CARTESIAN_POINT('Ctrl Pts',(0.408600000000001,-1.38664260250637,
1.26714345780971));
#22822=CARTESIAN_POINT('Ctrl Pts',(0.408600000000001,-1.34381660554335,
1.32516324902697));
#22823=CARTESIAN_POINT('Ctrl Pts',(0.408600000000001,-1.2978752047385,1.38066675809276));
#22824=CARTESIAN_POINT('Ctrl Pts',(0.408600000000001,-1.24906366160572,
1.43337782873043));
#22825=CARTESIAN_POINT('Ctrl Pts',(0.408600000000001,-1.20010611167173,
1.48624657057286));
#22826=CARTESIAN_POINT('Ctrl Pts',(0.408600000000001,-1.14826078782103,
1.53630714398619));
#22827=CARTESIAN_POINT('Ctrl Pts',(0.408600000000001,-1.09372545966621,
1.58326466535508));
#22828=CARTESIAN_POINT('Ctrl Pts',(0.408600000000001,-1.04029917410998,
1.62926724809456));
#22829=CARTESIAN_POINT('Ctrl Pts',(0.408600000000001,-0.984290607373418,
1.67229256006689));
#22830=CARTESIAN_POINT('Ctrl Pts',(0.408600000000001,-0.925845826339396,
1.71203418993537));
#22831=CARTESIAN_POINT('Ctrl Pts',(0.408600000000001,-0.904722483940492,
1.72639776595277));
#22832=CARTESIAN_POINT('Ctrl Pts',(0.408600000000001,-0.883280563501835,
1.74033206113498));
#22833=CARTESIAN_POINT('Ctrl Pts',(0.408600000000001,-0.861525859670525,
1.75382131162755));
#22834=CARTESIAN_POINT('Ctrl Pts',(0.4086,-0.905313301390919,-1.26710934922959));
#22835=CARTESIAN_POINT('Ctrl Pts',(0.440267204313647,-0.544607602467862,
-1.52079487885496));
#22836=CARTESIAN_POINT('Ctrl Pts',(0.508053930317628,0.473656038592629,
-1.7274214708134));
#22837=CARTESIAN_POINT('Ctrl Pts',(0.611960178011943,1.70289301291901,-0.651599460365548));
#22838=CARTESIAN_POINT('Ctrl Pts',(0.720318743082945,1.49728705490344,1.04067255962924));
#22839=CARTESIAN_POINT('Ctrl Pts',(0.828677308153947,-0.0167383245662881,
1.8231374532372));
#22840=CARTESIAN_POINT('Ctrl Pts',(0.922789802327533,-1.31892467005291,
1.11946232060462));
#22841=CARTESIAN_POINT('Ctrl Pts',(0.980782774810785,-1.55224362360984,
0.305528304683677));
#22842=CARTESIAN_POINT('Ctrl Pts',(1.0026562256037,-1.55363103362015,-0.000732727065787947));
#22843=CARTESIAN_POINT('Origin',(0.408600000000001,-2.59090492670967E-16,
0.));
#22844=CARTESIAN_POINT('',(0.408600000000001,-1.954,-2.39295984553393E-16));
#22845=CARTESIAN_POINT('Origin',(0.408600000000001,0.,0.));
#22846=CARTESIAN_POINT('Origin',(0.408600000000001,0.,0.));
#22847=CARTESIAN_POINT('',(0.408600000000001,0.90360677865021,-1.26612599672283));
#22848=CARTESIAN_POINT('Ctrl Pts',(0.408600000000001,0.863439746847563,
1.75538915071904));
#22849=CARTESIAN_POINT('Ctrl Pts',(0.408600000000001,0.923415504740013,
1.71873542152767));
#22850=CARTESIAN_POINT('Ctrl Pts',(0.4086,0.981160814141446,1.67880083042132));
#22851=CARTESIAN_POINT('Ctrl Pts',(0.408600000000001,1.03634589654915,1.63558766289775));
#22852=CARTESIAN_POINT('Ctrl Pts',(0.408600000000001,1.04229457843093,1.63092949486599));
#22853=CARTESIAN_POINT('Ctrl Pts',(0.408600000000001,1.04821347525907,1.6262331953884));
#22854=CARTESIAN_POINT('Ctrl Pts',(0.408600000000001,1.05410214691338,1.62149874228353));
#22855=CARTESIAN_POINT('Ctrl Pts',(0.408600000000001,1.11227764689379,1.5747260246523));
#22856=CARTESIAN_POINT('Ctrl Pts',(0.408600000000001,1.16750758234271,1.52423185527925));
#22857=CARTESIAN_POINT('Ctrl Pts',(0.408600000000001,1.21960503748186,1.4703938799972));
#22858=CARTESIAN_POINT('Ctrl Pts',(0.408600000000001,1.2316695712854,1.45792628304896));
#22859=CARTESIAN_POINT('Ctrl Pts',(0.408600000000001,1.2435658880977,1.44527926143554));
#22860=CARTESIAN_POINT('Ctrl Pts',(0.408600000000001,1.25529124126781,1.43245734592917));
#22861=CARTESIAN_POINT('Ctrl Pts',(0.408600000000001,1.26456542187468,1.42231583817185));
#22862=CARTESIAN_POINT('Ctrl Pts',(0.408600000000001,1.27372629854108,1.41207184696792));
#22863=CARTESIAN_POINT('Ctrl Pts',(0.408600000000001,1.28277244563777,1.40172855991044));
#22864=CARTESIAN_POINT('Ctrl Pts',(0.408600000000001,1.32967857189279,1.34809649717428));
#22865=CARTESIAN_POINT('Ctrl Pts',(0.408600000000001,1.37350887723089,1.29179113201222));
#22866=CARTESIAN_POINT('Ctrl Pts',(0.408600000000001,1.41411628391085,1.2331541048561));
#22867=CARTESIAN_POINT('Ctrl Pts',(0.408600000000001,1.44423515830919,1.18966250072767));
#22868=CARTESIAN_POINT('Ctrl Pts',(0.408600000000001,1.47258011132439,1.14488745049006));
#22869=CARTESIAN_POINT('Ctrl Pts',(0.408600000000001,1.4990734647959,1.0989628031704));
#22870=CARTESIAN_POINT('Ctrl Pts',(0.408600000000001,1.50943070523876,1.08100914490457));
#22871=CARTESIAN_POINT('Ctrl Pts',(0.4086,1.51950479225154,1.06287976458426));
#22872=CARTESIAN_POINT('Ctrl Pts',(0.4086,1.52929041576869,1.04458260423572));
#22873=CARTESIAN_POINT('Ctrl Pts',(0.4086,1.5370977611374,1.0299844286716));
#22874=CARTESIAN_POINT('Ctrl Pts',(0.408600000000001,1.54472327691443,1.01527558260098));
#22875=CARTESIAN_POINT('Ctrl Pts',(0.408600000000001,1.55215185596123,1.00048533214757));
#22876=CARTESIAN_POINT('Ctrl Pts',(0.408600000000001,1.58339919357882,0.938272095072908));
#22877=CARTESIAN_POINT('Ctrl Pts',(0.408600000000001,1.61121027972009,0.87454102427181));
#22878=CARTESIAN_POINT('Ctrl Pts',(0.408600000000001,1.63544819515225,0.809608649754739));
#22879=CARTESIAN_POINT('Ctrl Pts',(0.408600000000001,1.65914878364041,0.746115751931282));
#22880=CARTESIAN_POINT('Ctrl Pts',(0.408600000000001,1.67943295454144,0.681473222428096));
#22881=CARTESIAN_POINT('Ctrl Pts',(0.408600000000001,1.69612435377567,0.61597116125941));
#22882=CARTESIAN_POINT('Ctrl Pts',(0.408600000000001,1.70816660743026,0.568713742967382));
#22883=CARTESIAN_POINT('Ctrl Pts',(0.408600000000001,1.71833779962181,0.521008772156351));
#22884=CARTESIAN_POINT('Ctrl Pts',(0.408600000000001,1.72655511408715,0.472967494776519));
#22885=CARTESIAN_POINT('Ctrl Pts',(0.408600000000001,1.73065500678508,0.448998096603924));
#22886=CARTESIAN_POINT('Ctrl Pts',(0.408600000000001,1.73426828919771,0.424945031896326));
#22887=CARTESIAN_POINT('Ctrl Pts',(0.408600000000001,1.73738331488236,0.400822537981791));
#22888=CARTESIAN_POINT('Ctrl Pts',(0.408600000000001,1.73922474295558,0.386562675628391));
#22889=CARTESIAN_POINT('Ctrl Pts',(0.4086,1.74089203733157,0.372278557344402));
#22890=CARTESIAN_POINT('Ctrl Pts',(0.4086,1.74238263893657,0.357973186099987));
#22891=CARTESIAN_POINT('Ctrl Pts',(0.4086,1.74368858199248,0.345439991330694));
#22892=CARTESIAN_POINT('Ctrl Pts',(0.4086,1.74485804686663,0.332898075035613));
#22893=CARTESIAN_POINT('Ctrl Pts',(0.4086,1.74588926111498,0.320357474643566));
#22894=CARTESIAN_POINT('Ctrl Pts',(0.408600000000001,1.75123141071125,0.255391573107561));
#22895=CARTESIAN_POINT('Ctrl Pts',(0.408600000000001,1.7528745495965,0.19039258240519));
#22896=CARTESIAN_POINT('Ctrl Pts',(0.408600000000001,1.75066195802975,0.125627513646972));
#22897=CARTESIAN_POINT('Ctrl Pts',(0.408600000000001,1.74965524067005,0.0961597528542624));
#22898=CARTESIAN_POINT('Ctrl Pts',(0.408600000000001,1.74784961952587,0.0667405016615884));
#22899=CARTESIAN_POINT('Ctrl Pts',(0.408600000000001,1.74522680112737,0.0373956702521555));
#22900=CARTESIAN_POINT('Ctrl Pts',(0.408600000000001,1.73927155982219,-0.0292332477859586));
#22901=CARTESIAN_POINT('Ctrl Pts',(0.408600000000001,1.72910627580647,-0.0954804691698916));
#22902=CARTESIAN_POINT('Ctrl Pts',(0.408600000000001,1.71490485110609,-0.161032009093848));
#22903=CARTESIAN_POINT('Ctrl Pts',(0.408600000000001,1.70869172779967,-0.189710807810579));
#22904=CARTESIAN_POINT('Ctrl Pts',(0.408600000000001,1.70170546695327,-0.218256084698624));
#22905=CARTESIAN_POINT('Ctrl Pts',(0.408600000000001,1.69395810762654,-0.246639531074824));
#22906=CARTESIAN_POINT('Ctrl Pts',(0.408600000000001,1.68940335770069,-0.263326442682377));
#22907=CARTESIAN_POINT('Ctrl Pts',(0.408600000000001,1.68458551639814,-0.279957393553351));
#22908=CARTESIAN_POINT('Ctrl Pts',(0.408600000000001,1.67950681947972,-0.296526386780756));
#22909=CARTESIAN_POINT('Ctrl Pts',(0.408600000000001,1.67610525090757,-0.30762383314145));
#22910=CARTESIAN_POINT('Ctrl Pts',(0.408600000000001,1.67258631980131,-0.318694212312513));
#22911=CARTESIAN_POINT('Ctrl Pts',(0.408600000000001,1.6689560320264,-0.329720279574332));
#22912=CARTESIAN_POINT('Ctrl Pts',(0.408600000000001,1.6487117951502,-0.391206952615498));
#22913=CARTESIAN_POINT('Ctrl Pts',(0.408600000000001,1.62497416958449,-0.451433142841631));
#22914=CARTESIAN_POINT('Ctrl Pts',(0.408600000000001,1.59793571240631,-0.510129477960578));
#22915=CARTESIAN_POINT('Ctrl Pts',(0.408600000000001,1.57096028648465,-0.568688981908608));
#22916=CARTESIAN_POINT('Ctrl Pts',(0.408600000000001,1.54069864105028,-0.625726594487064));
#22917=CARTESIAN_POINT('Ctrl Pts',(0.408600000000001,1.50730181274075,-0.680942698188743));
#22918=CARTESIAN_POINT('Ctrl Pts',(0.408600000000001,1.4745521083011,-0.735088890149842));
#22919=CARTESIAN_POINT('Ctrl Pts',(0.408600000000001,1.43878678398125,-0.787484108438842));
#22920=CARTESIAN_POINT('Ctrl Pts',(0.408600000000001,1.40012093539101,-0.837804231710174));
#22921=CARTESIAN_POINT('Ctrl Pts',(0.408600000000001,1.39183183476257,-0.848591750428618));
#22922=CARTESIAN_POINT('Ctrl Pts',(0.408600000000001,1.38340935405792,-0.859283728160873));
#22923=CARTESIAN_POINT('Ctrl Pts',(0.408600000000001,1.37485451002538,-0.869876674256443));
#22924=CARTESIAN_POINT('Ctrl Pts',(0.408600000000001,1.36803642454044,-0.878319097255891));
#22925=CARTESIAN_POINT('Ctrl Pts',(0.408600000000001,1.36113760589381,-0.886694397807001));
#22926=CARTESIAN_POINT('Ctrl Pts',(0.408600000000001,1.35416372308826,-0.894995317810194));
#22927=CARTESIAN_POINT('Ctrl Pts',(0.408600000000001,1.31423588906621,-0.942520887906374));
#22928=CARTESIAN_POINT('Ctrl Pts',(0.408600000000001,1.27180173657993,-0.987671528671633));
#22929=CARTESIAN_POINT('Ctrl Pts',(0.408600000000001,1.22700455835745,-1.03018211725701));
#22930=CARTESIAN_POINT('Ctrl Pts',(0.408600000000001,1.1829959328827,-1.07194440332051));
#22931=CARTESIAN_POINT('Ctrl Pts',(0.408600000000001,1.13670602306087,-1.11115929871366));
#22932=CARTESIAN_POINT('Ctrl Pts',(0.408600000000001,1.08824736469086,-1.14753145000445));
#22933=CARTESIAN_POINT('Ctrl Pts',(0.408600000000001,1.04132560612878,-1.18275003340432));
#22934=CARTESIAN_POINT('Ctrl Pts',(0.408600000000001,0.992369867827824,
-1.2153036289198));
#22935=CARTESIAN_POINT('Ctrl Pts',(0.408600000000001,0.941469961039648,
-1.24487667804896));
#22936=CARTESIAN_POINT('Ctrl Pts',(0.408600000000001,0.928965840295594,
-1.2521416221405));
#22937=CARTESIAN_POINT('Ctrl Pts',(0.408600000000001,0.916344354236908,
-1.25922645029678));
#22938=CARTESIAN_POINT('Ctrl Pts',(0.408600000000001,0.903606778650211,
-1.26612599672283));
#22939=CARTESIAN_POINT('Origin',(0.408600000000001,0.,0.));
#22940=CARTESIAN_POINT('Origin',(-0.885456225603702,0.,0.));
#22941=CARTESIAN_POINT('Ctrl Pts',(0.408600000000001,0.903606778650209,
-1.26612599672283));
#22942=CARTESIAN_POINT('Ctrl Pts',(0.444719521690335,1.31409504259239,-0.973169388285302));
#22943=CARTESIAN_POINT('Ctrl Pts',(0.516958565071003,1.82250017258503,0.0372118057298887));
#22944=CARTESIAN_POINT('Ctrl Pts',(0.625317130142004,0.994051806197197,
1.52972919549323));
#22945=CARTESIAN_POINT('Ctrl Pts',(0.733675695213007,-0.703615338567789,
1.6815229998257));
#22946=CARTESIAN_POINT('Ctrl Pts',(0.813417909964438,-1.50026456430569,
0.713553299624354));
#22947=CARTESIAN_POINT('Ctrl Pts',(0.857040603025534,-1.55672331735519,
0.105986991352769));
#22948=CARTESIAN_POINT('Ctrl Pts',(0.864543774396297,-1.55583496332863,
0.00131431692112695));
#22949=CARTESIAN_POINT('Ctrl Pts',(0.178525917727935,1.13509973994375,-1.5904919303095));
#22950=CARTESIAN_POINT('Ctrl Pts',(0.214645439418269,1.65075005671844,-1.22248343600738));
#22951=CARTESIAN_POINT('Ctrl Pts',(0.286884482798937,2.28940233830353,0.046745013433751));
#22952=CARTESIAN_POINT('Ctrl Pts',(0.395243047869939,1.24871567297289,1.92162703181856));
#22953=CARTESIAN_POINT('Ctrl Pts',(0.50360161294094,-0.883872948609101,
2.11230854494337));
#22954=CARTESIAN_POINT('Ctrl Pts',(0.611960178011943,-2.2437405724288,0.459999581832252));
#22955=CARTESIAN_POINT('Ctrl Pts',(0.720318743082944,-1.64341174980208,
-1.59557661759511));
#22956=CARTESIAN_POINT('Ctrl Pts',(0.828677308153947,0.392945779374837,
-2.25633819105695));
#22957=CARTESIAN_POINT('Ctrl Pts',(0.937035873224949,2.08590841711691,-0.946028636835653));
#22958=CARTESIAN_POINT('Ctrl Pts',(1.04539443829595,1.95637548059159,1.19105133553842));
#22959=CARTESIAN_POINT('Ctrl Pts',(1.15375300336695,0.117472723211352,2.28736813879232));
#22960=CARTESIAN_POINT('Ctrl Pts',(1.26211156843795,-1.82406069577048,1.38518606320933));
#22961=CARTESIAN_POINT('Ctrl Pts',(1.37047013350896,-2.17185480860121,-0.727308039434555));
#22962=CARTESIAN_POINT('Ctrl Pts',(1.47882869857996,-0.622022654043615,
-2.20431378999848));
#22963=CARTESIAN_POINT('Ctrl Pts',(1.58718726365096,1.4712906547618,-1.75534285655934));
#22964=CARTESIAN_POINT('Ctrl Pts',(1.69554582872196,2.27908767273779,0.227335097164274));
#22965=CARTESIAN_POINT('Ctrl Pts',(1.80390439379297,1.09556770388087,2.01138046939323));
#22966=CARTESIAN_POINT('Ctrl Pts',(1.91226295886397,-1.04518727913395,2.03801522134292));
#22967=CARTESIAN_POINT('Ctrl Pts',(2.02062152393497,-2.27272600824398,0.283965628016336));
#22968=CARTESIAN_POINT('Ctrl Pts',(2.12898008900597,-1.51450731529388,-1.7181936614798));
#22969=CARTESIAN_POINT('Ctrl Pts',(2.23733865407697,0.56699002984457,-2.21910951530567));
#22970=CARTESIAN_POINT('Ctrl Pts',(2.34569721914798,2.15308520787897,-0.78111174266791));
#22971=CARTESIAN_POINT('Ctrl Pts',(2.45405578421898,1.85796319190442,1.33936666801838));
#22972=CARTESIAN_POINT('Ctrl Pts',(2.56241434928998,-0.0605379631590849,
2.28960105839));
#22973=CARTESIAN_POINT('Ctrl Pts',(2.67077291436098,-1.92611976024453,1.23932058494019));
#22974=CARTESIAN_POINT('Ctrl Pts',(2.77913147943199,-2.10883321481238,-0.893773336507565));
#22975=CARTESIAN_POINT('Ctrl Pts',(2.88749004450298,-0.448894737888299,
-2.24599145604085));
#22976=CARTESIAN_POINT('Ctrl Pts',(2.99584860957399,1.60308200591594,-1.63572506866501));
#22977=CARTESIAN_POINT('Ctrl Pts',(3.10420717464499,2.25472837895232,0.403567663658574));
#22978=CARTESIAN_POINT('Ctrl Pts',(3.21256573971599,0.93569695902205,2.0905603489318));
#22979=CARTESIAN_POINT('Ctrl Pts',(3.320924304787,-1.19965070554216,1.9503632900093));
#22980=CARTESIAN_POINT('Ctrl Pts',(3.42928286985799,-2.28920179463487,0.107221382123356));
#22981=CARTESIAN_POINT('Ctrl Pts',(3.537641434929,-1.37386884803431,-1.83194774797522));
#22982=CARTESIAN_POINT('Ctrl Pts',(3.60988047830967,0.0295369701314518,
-2.05391554560157));
#22983=CARTESIAN_POINT('Ctrl Pts',(3.646,0.629287956476874,-1.84989531266857));
#22984=CARTESIAN_POINT('Ctrl Pts',(0.25521727848529,1.05793541951257,-1.48236995244728));
#22985=CARTESIAN_POINT('Ctrl Pts',(0.291336800175624,1.53853171867642,-1.13937875343336));
#22986=CARTESIAN_POINT('Ctrl Pts',(0.363575843556292,2.13376828306403,0.0435672775324635));
#22987=CARTESIAN_POINT('Ctrl Pts',(0.471934408627294,1.16382771738099,1.79099441971012));
#22988=CARTESIAN_POINT('Ctrl Pts',(0.580292973698296,-0.823787078595329,
1.96871336323748));
#22989=CARTESIAN_POINT('Ctrl Pts',(0.688651538769298,-2.09121061369238,
0.428728712954709));
#22990=CARTESIAN_POINT('Ctrl Pts',(0.797010103840299,-1.53169227141652,
-1.48710898161564));
#22991=CARTESIAN_POINT('Ctrl Pts',(0.905368668911303,0.36623324217237,-2.10295184354139));
#22992=CARTESIAN_POINT('Ctrl Pts',(1.0137272339823,1.94410792168513,-0.881717409988328));
#22993=CARTESIAN_POINT('Ctrl Pts',(1.12208579905331,1.82338066158515,1.11008341380316));
#22994=CARTESIAN_POINT('Ctrl Pts',(1.23044436412431,0.109486902638216,2.13187236886589));
#22995=CARTESIAN_POINT('Ctrl Pts',(1.33880292919531,-1.70006066382498,1.29102082162132));
#22996=CARTESIAN_POINT('Ctrl Pts',(1.44716149426631,-2.02421165929592,-0.677865485064943));
#22997=CARTESIAN_POINT('Ctrl Pts',(1.55552005933731,-0.579737422444096,
-2.0544640722717));
#22998=CARTESIAN_POINT('Ctrl Pts',(1.66387862440832,1.37127200482619,-1.63601427785942));
#22999=CARTESIAN_POINT('Ctrl Pts',(1.77223718947932,2.12415481064533,0.211880809170421));
#23000=CARTESIAN_POINT('Ctrl Pts',(1.88059575455032,1.02109077962353,1.87464639961275));
#23001=CARTESIAN_POINT('Ctrl Pts',(1.98895431962132,-0.974135226807976,
1.89947051549079));
#23002=CARTESIAN_POINT('Ctrl Pts',(2.09731288469232,-2.11822561344951,0.264661584555997));
#23003=CARTESIAN_POINT('Ctrl Pts',(2.20567144976332,-1.41155078763359,-1.60139049291963));
#23004=CARTESIAN_POINT('Ctrl Pts',(2.31403001483433,0.528445927679258,-2.06825398104274));
#23005=CARTESIAN_POINT('Ctrl Pts',(2.42238857990533,2.00671802000115,-0.728011601171293));
#23006=CARTESIAN_POINT('Ctrl Pts',(2.53074714497633,1.73165846110027,1.24831623860771));
#23007=CARTESIAN_POINT('Ctrl Pts',(2.63910571004733,-0.0564225796178219,
2.13395349411699));
#23008=CARTESIAN_POINT('Ctrl Pts',(2.74746427511834,-1.79518173150733,1.15507130942012));
#23009=CARTESIAN_POINT('Ctrl Pts',(2.85582284018934,-1.96547428678394,-0.833014436030208));
#23010=CARTESIAN_POINT('Ctrl Pts',(2.96418140526034,-0.418378778651093,
-2.09330848176036));
#23011=CARTESIAN_POINT('Ctrl Pts',(3.07253997033134,1.49410415205079,-1.52452813248913));
#23012=CARTESIAN_POINT('Ctrl Pts',(3.18089853540234,2.10145146680416,0.376133048515631));
#23013=CARTESIAN_POINT('Ctrl Pts',(3.28925710047335,0.872088081817974,1.94844361419121));
#23014=CARTESIAN_POINT('Ctrl Pts',(3.39761566554435,-1.11809819681501,1.81777718099042));
#23015=CARTESIAN_POINT('Ctrl Pts',(3.50597423061535,-2.13358137239638,0.0999324498858656));
#23016=CARTESIAN_POINT('Ctrl Pts',(3.61433279568635,-1.28047295312785,-1.70741155255248));
#23017=CARTESIAN_POINT('Ctrl Pts',(3.68657183906702,0.027529040653905,-1.91428993234292));
#23018=CARTESIAN_POINT('Ctrl Pts',(3.72269136075735,0.5865088280811,-1.72413903800149));
#23019=CARTESIAN_POINT('Ctrl Pts',(0.331908639242645,0.98077109908139,-1.37424797458505));
#23020=CARTESIAN_POINT('Ctrl Pts',(0.368028160932979,1.42631338063441,-1.05627407085933));
#23021=CARTESIAN_POINT('Ctrl Pts',(0.440267204313648,1.97813422782453,0.0403895416311738));
#23022=CARTESIAN_POINT('Ctrl Pts',(0.548625769384648,1.07893976178909,1.66036180760168));
#23023=CARTESIAN_POINT('Ctrl Pts',(0.656984334455652,-0.763701208581558,
1.82511818153158));
#23024=CARTESIAN_POINT('Ctrl Pts',(0.765342899526653,-1.93868065495597,
0.39745784407717));
#23025=CARTESIAN_POINT('Ctrl Pts',(0.873701464597655,-1.41997279303096,
-1.37864134563618));
#23026=CARTESIAN_POINT('Ctrl Pts',(0.982060029668658,0.339520704969898,
-1.94956549602583));
#23027=CARTESIAN_POINT('Ctrl Pts',(1.09041859473966,1.80230742625336,-0.817406183141006));
#23028=CARTESIAN_POINT('Ctrl Pts',(1.19877715981066,1.69038584257871,1.02911549206791));
#23029=CARTESIAN_POINT('Ctrl Pts',(1.30713572488166,0.101501082065082,1.97637659893946));
#23030=CARTESIAN_POINT('Ctrl Pts',(1.41549428995266,-1.57606063187948,1.19685558003331));
#23031=CARTESIAN_POINT('Ctrl Pts',(1.52385285502367,-1.87656850999063,-0.62842293069533));
#23032=CARTESIAN_POINT('Ctrl Pts',(1.63221142009467,-0.537452190844577,
-1.90461435454492));
#23033=CARTESIAN_POINT('Ctrl Pts',(1.74056998516567,1.27125335489057,-1.51668569915951));
#23034=CARTESIAN_POINT('Ctrl Pts',(1.84892855023667,1.96922194855287,0.19642652117657));
#23035=CARTESIAN_POINT('Ctrl Pts',(1.95728711530767,0.946613855366191,1.73791232983226));
#23036=CARTESIAN_POINT('Ctrl Pts',(2.06564568037868,-0.903083174482,1.76092580963867));
#23037=CARTESIAN_POINT('Ctrl Pts',(2.17400424544968,-1.96372521865503,0.245357541095656));
#23038=CARTESIAN_POINT('Ctrl Pts',(2.28236281052068,-1.3085942599733,-1.48458732435947));
#23039=CARTESIAN_POINT('Ctrl Pts',(2.39072137559169,0.489901825513946,-1.91739844677981));
#23040=CARTESIAN_POINT('Ctrl Pts',(2.49907994066268,1.86035083212334,-0.674911459674677));
#23041=CARTESIAN_POINT('Ctrl Pts',(2.60743850573369,1.60535373029612,1.15726580919705));
#23042=CARTESIAN_POINT('Ctrl Pts',(2.71579707080469,-0.0523071960765568,
1.97830592984397));
#23043=CARTESIAN_POINT('Ctrl Pts',(2.82415563587569,-1.66424370277014,1.07082203390004));
#23044=CARTESIAN_POINT('Ctrl Pts',(2.9325142009467,-1.8221153587555,-0.772255535552851));
#23045=CARTESIAN_POINT('Ctrl Pts',(3.04087276601769,-0.387862819413889,
-1.94062550747986));
#23046=CARTESIAN_POINT('Ctrl Pts',(3.1492313310887,1.38512629818565,-1.41333119631325));
#23047=CARTESIAN_POINT('Ctrl Pts',(3.2575898961597,1.948174554656,0.348698433372686));
#23048=CARTESIAN_POINT('Ctrl Pts',(3.3659484612307,0.808479204613899,1.80632687945063));
#23049=CARTESIAN_POINT('Ctrl Pts',(3.47430702630171,-1.03654568808786,1.68519107197153));
#23050=CARTESIAN_POINT('Ctrl Pts',(3.5826655913727,-1.9779609501579,0.0926435176483781));
#23051=CARTESIAN_POINT('Ctrl Pts',(3.69102415644371,-1.18707705822139,-1.58287535712974));
#23052=CARTESIAN_POINT('Ctrl Pts',(3.76326319982438,0.0255211111763578,
-1.77466431908426));
#23053=CARTESIAN_POINT('Ctrl Pts',(3.79938272151471,0.543729699685325,-1.59838276333441));
#23054=CARTESIAN_POINT('Ctrl Pts',(0.408600000000001,0.903606778650209,
-1.26612599672283));
#23055=CARTESIAN_POINT('Ctrl Pts',(0.444719521690335,1.31409504259239,-0.973169388285302));
#23056=CARTESIAN_POINT('Ctrl Pts',(0.516958565071003,1.82250017258503,0.0372118057298887));
#23057=CARTESIAN_POINT('Ctrl Pts',(0.625317130142004,0.994051806197197,
1.52972919549323));
#23058=CARTESIAN_POINT('Ctrl Pts',(0.733675695213007,-0.703615338567789,
1.6815229998257));
#23059=CARTESIAN_POINT('Ctrl Pts',(0.842034260284009,-1.78615069621955,
0.366186975199626));
#23060=CARTESIAN_POINT('Ctrl Pts',(0.95039282535501,-1.30825331464541,-1.27017370965671));
#23061=CARTESIAN_POINT('Ctrl Pts',(1.05875139042601,0.312808167767432,-1.79617914851027));
#23062=CARTESIAN_POINT('Ctrl Pts',(1.16710995549701,1.66050693082158,-0.753094956293683));
#23063=CARTESIAN_POINT('Ctrl Pts',(1.27546852056802,1.55739102357227,0.948147570332657));
#23064=CARTESIAN_POINT('Ctrl Pts',(1.38382708563902,0.093515261491943,1.82088082901303));
#23065=CARTESIAN_POINT('Ctrl Pts',(1.49218565071002,-1.45206059993398,1.1026903384453));
#23066=CARTESIAN_POINT('Ctrl Pts',(1.60054421578102,-1.72892536068535,-0.57898037632572));
#23067=CARTESIAN_POINT('Ctrl Pts',(1.70890278085203,-0.495166959245057,
-1.75476463681813));
#23068=CARTESIAN_POINT('Ctrl Pts',(1.81726134592303,1.17123470495496,-1.39735712045959));
#23069=CARTESIAN_POINT('Ctrl Pts',(1.92561991099403,1.81428908646041,0.180972233182718));
#23070=CARTESIAN_POINT('Ctrl Pts',(2.03397847606503,0.872136931108851,1.60117826005178));
#23071=CARTESIAN_POINT('Ctrl Pts',(2.14233704113603,-0.832031122156023,
1.62238110378654));
#23072=CARTESIAN_POINT('Ctrl Pts',(2.25069560620703,-1.80922482386055,0.226053497635316));
#23073=CARTESIAN_POINT('Ctrl Pts',(2.35905417127804,-1.20563773231302,-1.3677841557993));
#23074=CARTESIAN_POINT('Ctrl Pts',(2.46741273634904,0.451357723348635,-1.76654291251687));
#23075=CARTESIAN_POINT('Ctrl Pts',(2.57577130142004,1.71398364424552,-0.621811318178061));
#23076=CARTESIAN_POINT('Ctrl Pts',(2.68412986649104,1.47904899949198,1.06621537978638));
#23077=CARTESIAN_POINT('Ctrl Pts',(2.79248843156204,-0.0481918125352924,
1.82265836557096));
#23078=CARTESIAN_POINT('Ctrl Pts',(2.90084699663305,-1.53330567403294,0.98657275837997));
#23079=CARTESIAN_POINT('Ctrl Pts',(3.00920556170405,-1.67875643072706,-0.711496635075496));
#23080=CARTESIAN_POINT('Ctrl Pts',(3.11756412677505,-0.357346860176684,
-1.78794253319936));
#23081=CARTESIAN_POINT('Ctrl Pts',(3.22592269184605,1.2761484443205,-1.30213426013737));
#23082=CARTESIAN_POINT('Ctrl Pts',(3.33428125691706,1.79489764250785,0.32126381822974));
#23083=CARTESIAN_POINT('Ctrl Pts',(3.44263982198805,0.744870327409823,1.66421014471004));
#23084=CARTESIAN_POINT('Ctrl Pts',(3.55099838705906,-0.954993179360717,
1.55260496295264));
#23085=CARTESIAN_POINT('Ctrl Pts',(3.65935695213006,-1.82234052791941,0.0853545854108896));
#23086=CARTESIAN_POINT('Ctrl Pts',(3.76771551720107,-1.09368116331493,-1.45833916170699));
#23087=CARTESIAN_POINT('Ctrl Pts',(3.83995456058173,0.0235131816988109,
-1.63503870582561));
#23088=CARTESIAN_POINT('Ctrl Pts',(3.87607408227207,0.50095057128955,-1.47262648866733));
#23089=CARTESIAN_POINT('Ctrl Pts',(3.646,0.629287956476874,-1.84989531266857));
#23090=CARTESIAN_POINT('Ctrl Pts',(3.60988047830967,0.0295369701314485,
-2.05391554560157));
#23091=CARTESIAN_POINT('Ctrl Pts',(3.57376095661933,-0.672165938951437,
-1.9429316467884));
#23092=CARTESIAN_POINT('Ctrl Pts',(3.537641434929,-1.17557288459297,-1.56424484236538));
#23093=CARTESIAN_POINT('Ctrl Pts',(3.50325085399408,-1.65488314389577,-1.20368471900189));
#23094=CARTESIAN_POINT('Ctrl Pts',(3.46886027305915,-1.95442683952169,-0.600436693209037));
#23095=CARTESIAN_POINT('Ctrl Pts',(3.43446969212423,-1.95694215816793,0.000613609334558611));
#23096=CARTESIAN_POINT('Origin',(1.705,0.,0.));
#23097=CARTESIAN_POINT('',(1.4,0.,0.));
#23098=CARTESIAN_POINT('',(2.,-0.98360655737705,1.20457062211215E-16));
#23099=CARTESIAN_POINT('',(1.705,-0.5,-6.12323399573677E-17));
#23100=CARTESIAN_POINT('Origin',(2.,0.,0.));
#23101=CARTESIAN_POINT('Origin',(2.,7.07050159149938E-17,1.15470053837925));
#23102=CARTESIAN_POINT('',(4.,-1.,0.577350269189626));
#23103=CARTESIAN_POINT('',(4.,7.07050159149938E-17,1.15470053837925));
#23104=CARTESIAN_POINT('',(4.,-0.25,1.01036297108185));
#23105=CARTESIAN_POINT('',(2.,-1.,0.577350269189626));
#23106=CARTESIAN_POINT('',(2.,-1.,0.577350269189626));
#23107=CARTESIAN_POINT('',(2.,7.07050159149938E-17,1.15470053837925));
#23108=CARTESIAN_POINT('',(2.,7.07050159149938E-17,1.15470053837925));
#23109=CARTESIAN_POINT('',(2.,7.07050159149938E-17,1.15470053837925));
#23110=CARTESIAN_POINT('Origin',(2.,1.,0.577350269189626));
#23111=CARTESIAN_POINT('',(4.,1.,0.577350269189626));
#23112=CARTESIAN_POINT('',(4.,0.75,0.721687836487032));
#23113=CARTESIAN_POINT('',(2.,1.,0.577350269189626));
#23114=CARTESIAN_POINT('',(2.,1.,0.577350269189626));
#23115=CARTESIAN_POINT('',(2.,1.,0.577350269189626));
#23116=CARTESIAN_POINT('Origin',(2.,1.,-0.577350269189626));
#23117=CARTESIAN_POINT('',(4.,1.,-0.577350269189626));
#23118=CARTESIAN_POINT('',(4.,1.,-0.288675134594813));
#23119=CARTESIAN_POINT('',(2.,1.,-0.577350269189626));
#23120=CARTESIAN_POINT('',(2.,1.,-0.577350269189626));
#23121=CARTESIAN_POINT('',(2.,1.,-0.577350269189626));
#23122=CARTESIAN_POINT('Origin',(2.,-2.12115047744981E-16,-1.15470053837925));
#23123=CARTESIAN_POINT('',(4.,-2.12115047744981E-16,-1.15470053837925));
#23124=CARTESIAN_POINT('',(4.,0.25,-1.01036297108185));
#23125=CARTESIAN_POINT('',(2.,-2.12115047744981E-16,-1.15470053837925));
#23126=CARTESIAN_POINT('',(2.,-2.12115047744981E-16,-1.15470053837925));
#23127=CARTESIAN_POINT('',(2.,-2.12115047744981E-16,-1.15470053837925));
#23128=CARTESIAN_POINT('Origin',(2.,-1.,-0.577350269189626));
#23129=CARTESIAN_POINT('',(4.,-1.,-0.577350269189626));
#23130=CARTESIAN_POINT('',(4.,-0.75,-0.721687836487032));
#23131=CARTESIAN_POINT('',(2.,-1.,-0.577350269189626));
#23132=CARTESIAN_POINT('',(2.,-1.,-0.577350269189626));
#23133=CARTESIAN_POINT('',(2.,-1.,-0.577350269189626));
#23134=CARTESIAN_POINT('Origin',(2.,-1.,0.577350269189626));
#23135=CARTESIAN_POINT('',(4.,-1.,0.288675134594813));
#23136=CARTESIAN_POINT('',(2.,-1.,0.577350269189626));
#23137=CARTESIAN_POINT('Origin',(2.,0.,0.));
#23138=CARTESIAN_POINT('Origin',(0.,1.5,0.));
#23139=CARTESIAN_POINT('',(1.04083408558608E-16,-1.5,-1.83697019872103E-16));
#23140=CARTESIAN_POINT('Origin',(0.,0.,0.));
#23141=CARTESIAN_POINT('Origin',(0.225,0.,0.));
#23142=CARTESIAN_POINT('',(0.225,-1.75,-2.14313189850787E-16));
#23143=CARTESIAN_POINT('Origin',(2.025,0.,0.));
#23144=CARTESIAN_POINT('Origin',(3.646,0.,0.));
#23145=CARTESIAN_POINT('Origin',(3.8,0.,0.));
#23146=CARTESIAN_POINT('',(4.,-1.6,-1.95943487863577E-16));
#23147=CARTESIAN_POINT('Origin',(4.,0.,0.));
#23148=CARTESIAN_POINT('',(3.8,-1.8,-2.20436423846524E-16));
#23149=CARTESIAN_POINT('Origin',(4.,0.,0.));
#23240=UNCERTAINTY_MEASURE_WITH_UNIT(LENGTH_MEASURE(0.01),#23255,
'DISTANCE_ACCURACY_VALUE',
'Maximum model space distance between geometric entities at asserted c
onnectivities');
#23242=UNCERTAINTY_MEASURE_WITH_UNIT(LENGTH_MEASURE(0.01),#23255,
'DISTANCE_ACCURACY_VALUE',
'Maximum model space distance between geometric entities at asserted c
onnectivities');
#23252=(
GEOMETRIC_REPRESENTATION_CONTEXT(3)
GLOBAL_UNCERTAINTY_ASSIGNED_CONTEXT((#23240))
GLOBAL_UNIT_ASSIGNED_CONTEXT((#23255,#23257,#23258))
REPRESENTATION_CONTEXT('','3D')
);
#23254=(
GEOMETRIC_REPRESENTATION_CONTEXT(3)
GLOBAL_UNCERTAINTY_ASSIGNED_CONTEXT((#23242))
GLOBAL_UNIT_ASSIGNED_CONTEXT((#23255,#23257,#23258))
REPRESENTATION_CONTEXT('','3D')
);
#23255=(
LENGTH_UNIT()
NAMED_UNIT(*)
SI_UNIT(.MILLI.,.METRE.)
);
#23257=(
NAMED_UNIT(*)
PLANE_ANGLE_UNIT()
SI_UNIT($,.RADIAN.)
);
#23258=(
NAMED_UNIT(*)
SI_UNIT($,.STERADIAN.)
SOLID_ANGLE_UNIT()
);
#23268=SHAPE_DEFINITION_REPRESENTATION(#23279,#23308);
#23279=PRODUCT_DEFINITION_SHAPE('',$,#23320);
#23308=SHAPE_REPRESENTATION('',(#7755),#23252);
#23310=PRODUCT_DEFINITION_CONTEXT('part definition',#23345,'design');
#23320=PRODUCT_DEFINITION('2026-10-11-09-11-55-273',
'09_ISO_4026_M4x4_Set_Screw',#23331,#23310);
#23331=PRODUCT_DEFINITION_FORMATION('',$,#23356);
#23345=APPLICATION_CONTEXT(
'Core Data for Automotive Mechanical Design Process');
#23346=PRODUCT_CONTEXT('part definition',#23345,'mechanical');
#23356=PRODUCT('2026-10-11-09-11-55-273','09_ISO_4026_M4x4_Set_Screw',$,
(#23346));
#23463=COLOUR_RGB('Black',0.12,0.14,0.17);
#23464=FILL_AREA_STYLE_COLOUR('',#23463);
#23465=FILL_AREA_STYLE('',(#23464));
#23466=SURFACE_STYLE_FILL_AREA(#23465);
#23467=SURFACE_SIDE_STYLE('',(#23466));
#23468=SURFACE_STYLE_USAGE(.BOTH.,#23467);
#23469=PRESENTATION_STYLE_ASSIGNMENT((#23468));
ENDSEC;
END-ISO-10303-21;
